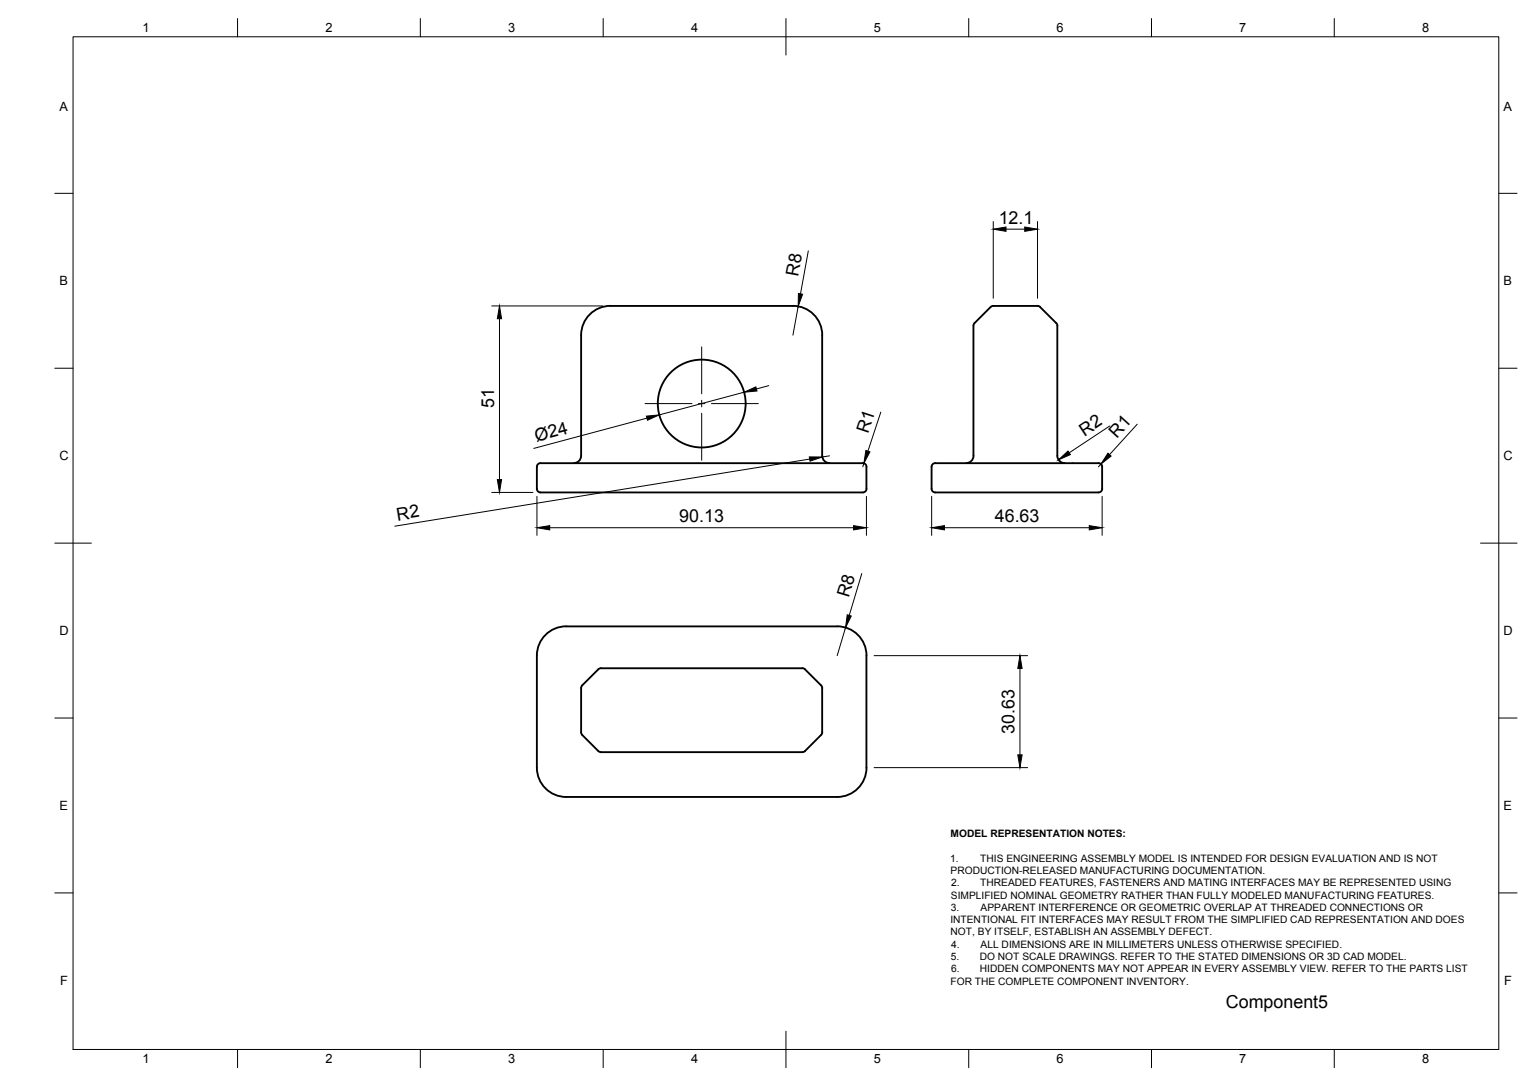
ISO-10303-21;
HEADER;
/* Generated by software containing ST-Developer
 * from STEP Tools, Inc. (www.steptools.com) 
 */

FILE_DESCRIPTION(
/* description */ ('STEP AP214'),
/* implementation_level */ '2;1');

FILE_NAME(
/* name */ 'Component5.step',
/* time_stamp */ '2026-10-06T11:02:40-07:00',
/* author */ (''),
/* organization */ (''),
/* preprocessor_version */ 'ST-DEVELOPER v20.2',
/* originating_system */ 'Autodesk Translation Framework v15.15.0.0',
/* authorisation */ '');

FILE_SCHEMA (('AUTOMOTIVE_DESIGN { 1 0 10303 214 3 1 1 }'));
ENDSEC;

DATA;
#10=MECHANICAL_DESIGN_GEOMETRIC_PRESENTATION_REPRESENTATION('',(#2940),#130910);
#78=CONICAL_SURFACE('',#48628,2.99999999999998,0.78539816339745);
#79=CONICAL_SURFACE('',#48632,2.99999999999998,0.78539816339745);
#80=CONICAL_SURFACE('',#48637,3.00000000000006,0.785398163397453);
#81=CONICAL_SURFACE('',#48641,3.00000000000006,0.785398163397453);
#721=FACE_BOUND('',#15164,.T.);
#722=FACE_BOUND('',#15172,.T.);
#723=FACE_BOUND('',#15175,.T.);
#2924=SHAPE_REPRESENTATION_RELATIONSHIP('SRR','None',#130946,#2932);
#2932=ADVANCED_BREP_SHAPE_REPRESENTATION('',(#2946),#130906);
#2940=STYLED_ITEM('',(#130991),#2946);
#2946=MANIFOLD_SOLID_BREP('Body1',#45456);
#3618=PLANE('',#48578);
#3619=PLANE('',#48591);
#3620=PLANE('',#48592);
#3621=PLANE('',#48593);
#3622=PLANE('',#48594);
#3623=PLANE('',#48595);
#3624=PLANE('',#48600);
#3625=PLANE('',#48601);
#3626=PLANE('',#48604);
#3627=PLANE('',#48605);
#3628=PLANE('',#48608);
#3629=PLANE('',#48627);
#3630=PLANE('',#48631);
#3631=PLANE('',#48635);
#3632=PLANE('',#48636);
#3633=PLANE('',#48640);
#3634=PLANE('',#48644);
#5186=LINE('',#96931,#6960);
#5187=LINE('',#96938,#6961);
#5188=LINE('',#96942,#6962);
#5189=LINE('',#96946,#6963);
#5190=LINE('',#96949,#6964);
#5191=LINE('',#96952,#6965);
#5192=LINE('',#96956,#6966);
#5193=LINE('',#96960,#6967);
#5194=LINE('',#96964,#6968);
#5195=LINE('',#96968,#6969);
#5196=LINE('',#96972,#6970);
#5197=LINE('',#96976,#6971);
#5198=LINE('',#96980,#6972);
#5199=LINE('',#96985,#6973);
#5200=LINE('',#96987,#6974);
#5201=LINE('',#96989,#6975);
#5202=LINE('',#96990,#6976);
#5203=LINE('',#96994,#6977);
#5204=LINE('',#96996,#6978);
#5205=LINE('',#96998,#6979);
#5206=LINE('',#96999,#6980);
#5207=LINE('',#97003,#6981);
#5208=LINE('',#97005,#6982);
#5209=LINE('',#97007,#6983);
#5210=LINE('',#97008,#6984);
#5211=LINE('',#97012,#6985);
#5212=LINE('',#97014,#6986);
#5213=LINE('',#97016,#6987);
#5214=LINE('',#97017,#6988);
#5215=LINE('',#97023,#6989);
#5216=LINE('',#97027,#6990);
#5217=LINE('',#97031,#6991);
#5218=LINE('',#97034,#6992);
#5219=LINE('',#97038,#6993);
#5220=LINE('',#97040,#6994);
#5221=LINE('',#97042,#6995);
#5222=LINE('',#97043,#6996);
#5223=LINE('',#97047,#6997);
#5224=LINE('',#97049,#6998);
#5225=LINE('',#97051,#6999);
#5226=LINE('',#97055,#7000);
#5227=LINE('',#97060,#7001);
#5228=LINE('',#97062,#7002);
#5229=LINE('',#97064,#7003);
#5230=LINE('',#97065,#7004);
#5231=LINE('',#97069,#7005);
#5232=LINE('',#97071,#7006);
#5233=LINE('',#97073,#7007);
#5234=LINE('',#97077,#7008);
#5235=LINE('',#97082,#7009);
#5236=LINE('',#97084,#7010);
#5237=LINE('',#97086,#7011);
#5238=LINE('',#97087,#7012);
#5239=LINE('',#97109,#7013);
#5240=LINE('',#97111,#7014);
#5241=LINE('',#97113,#7015);
#5242=LINE('',#97114,#7016);
#5243=LINE('',#97118,#7017);
#5244=LINE('',#97124,#7018);
#5245=LINE('',#97125,#7019);
#5246=LINE('',#97126,#7020);
#5247=LINE('',#97130,#7021);
#5248=LINE('',#97135,#7022);
#5249=LINE('',#97137,#7023);
#5250=LINE('',#97138,#7024);
#5251=LINE('',#97142,#7025);
#5252=LINE('',#97144,#7026);
#5253=LINE('',#97146,#7027);
#5254=LINE('',#97147,#7028);
#5255=LINE('',#97151,#7029);
#5256=LINE('',#97157,#7030);
#5257=LINE('',#97158,#7031);
#5258=LINE('',#97159,#7032);
#5259=LINE('',#97163,#7033);
#5260=LINE('',#97168,#7034);
#5261=LINE('',#97170,#7035);
#5262=LINE('',#97171,#7036);
#6960=VECTOR('',#58531,12.);
#6961=VECTOR('',#58538,1000.);
#6962=VECTOR('',#58541,1000.);
#6963=VECTOR('',#58544,1000.);
#6964=VECTOR('',#58547,1000.);
#6965=VECTOR('',#58548,1000.);
#6966=VECTOR('',#58551,1000.);
#6967=VECTOR('',#58554,1000.);
#6968=VECTOR('',#58557,1000.);
#6969=VECTOR('',#58560,1000.);
#6970=VECTOR('',#58563,1000.);
#6971=VECTOR('',#58566,1000.);
#6972=VECTOR('',#58569,1000.);
#6973=VECTOR('',#58574,1000.);
#6974=VECTOR('',#58575,1000.);
#6975=VECTOR('',#58576,1000.);
#6976=VECTOR('',#58577,1000.);
#6977=VECTOR('',#58580,1000.);
#6978=VECTOR('',#58581,1000.);
#6979=VECTOR('',#58582,1000.);
#6980=VECTOR('',#58583,1000.);
#6981=VECTOR('',#58586,1000.);
#6982=VECTOR('',#58587,1000.);
#6983=VECTOR('',#58588,1000.);
#6984=VECTOR('',#58589,1000.);
#6985=VECTOR('',#58592,1000.);
#6986=VECTOR('',#58593,1000.);
#6987=VECTOR('',#58594,1000.);
#6988=VECTOR('',#58595,1000.);
#6989=VECTOR('',#58600,1000.);
#6990=VECTOR('',#58603,1000.);
#6991=VECTOR('',#58606,1000.);
#6992=VECTOR('',#58609,1000.);
#6993=VECTOR('',#58612,1000.);
#6994=VECTOR('',#58613,1000.);
#6995=VECTOR('',#58614,1000.);
#6996=VECTOR('',#58615,1000.);
#6997=VECTOR('',#58618,1000.);
#6998=VECTOR('',#58619,1000.);
#6999=VECTOR('',#58620,1000.);
#7000=VECTOR('',#58623,1000.);
#7001=VECTOR('',#58628,1000.);
#7002=VECTOR('',#58629,1000.);
#7003=VECTOR('',#58630,1000.);
#7004=VECTOR('',#58631,1000.);
#7005=VECTOR('',#58634,1000.);
#7006=VECTOR('',#58635,1000.);
#7007=VECTOR('',#58636,1000.);
#7008=VECTOR('',#58639,1000.);
#7009=VECTOR('',#58644,1000.);
#7010=VECTOR('',#58645,1000.);
#7011=VECTOR('',#58646,1000.);
#7012=VECTOR('',#58647,1000.);
#7013=VECTOR('',#58686,1000.);
#7014=VECTOR('',#58687,1000.);
#7015=VECTOR('',#58688,1000.);
#7016=VECTOR('',#58689,1000.);
#7017=VECTOR('',#58692,1000.);
#7018=VECTOR('',#58699,1000.);
#7019=VECTOR('',#58700,1000.);
#7020=VECTOR('',#58701,1000.);
#7021=VECTOR('',#58704,1000.);
#7022=VECTOR('',#58711,1000.);
#7023=VECTOR('',#58712,1000.);
#7024=VECTOR('',#58713,1000.);
#7025=VECTOR('',#58716,1000.);
#7026=VECTOR('',#58717,1000.);
#7027=VECTOR('',#58718,1000.);
#7028=VECTOR('',#58719,1000.);
#7029=VECTOR('',#58722,1000.);
#7030=VECTOR('',#58729,1000.);
#7031=VECTOR('',#58730,1000.);
#7032=VECTOR('',#58731,1000.);
#7033=VECTOR('',#58734,1000.);
#7034=VECTOR('',#58741,1000.);
#7035=VECTOR('',#58742,1000.);
#7036=VECTOR('',#58743,1000.);
#8619=CYLINDRICAL_SURFACE('',#48575,12.);
#8620=CYLINDRICAL_SURFACE('',#48609,8.00000000000001);
#8621=CYLINDRICAL_SURFACE('',#48612,8.00000000000001);
#8622=CYLINDRICAL_SURFACE('',#48615,8.);
#8623=CYLINDRICAL_SURFACE('',#48618,8.);
#8624=CYLINDRICAL_SURFACE('',#48621,8.);
#8625=CYLINDRICAL_SURFACE('',#48624,8.);
#8626=CYLINDRICAL_SURFACE('',#48645,1.);
#8627=CYLINDRICAL_SURFACE('',#48652,1.);
#8628=CYLINDRICAL_SURFACE('',#48654,1.);
#8629=CYLINDRICAL_SURFACE('',#48660,1.);
#8630=CYLINDRICAL_SURFACE('',#48661,1.);
#8631=CYLINDRICAL_SURFACE('',#48668,1.);
#8632=CYLINDRICAL_SURFACE('',#48670,1.);
#8633=CYLINDRICAL_SURFACE('',#48676,1.);
#8634=CYLINDRICAL_SURFACE('',#48677,1.);
#8635=CYLINDRICAL_SURFACE('',#48682,1.);
#8636=CYLINDRICAL_SURFACE('',#48686,1.);
#8637=CYLINDRICAL_SURFACE('',#48688,1.);
#8638=CYLINDRICAL_SURFACE('',#48693,1.);
#8639=CYLINDRICAL_SURFACE('',#48697,1.);
#8640=CYLINDRICAL_SURFACE('',#48699,1.);
#8641=CYLINDRICAL_SURFACE('',#48704,1.);
#8642=CYLINDRICAL_SURFACE('',#48708,1.);
#8643=CYLINDRICAL_SURFACE('',#48710,1.);
#8644=CYLINDRICAL_SURFACE('',#48715,1.);
#8645=CYLINDRICAL_SURFACE('',#48719,1.);
#8646=CYLINDRICAL_SURFACE('',#48724,1.99999999999999);
#8647=CYLINDRICAL_SURFACE('',#48726,2.);
#8648=CYLINDRICAL_SURFACE('',#48732,2.);
#8649=CYLINDRICAL_SURFACE('',#48734,1.99999999999999);
#8650=CYLINDRICAL_SURFACE('',#48740,1.99999999999999);
#8651=CYLINDRICAL_SURFACE('',#48742,2.);
#8652=CYLINDRICAL_SURFACE('',#48748,2.);
#8653=CYLINDRICAL_SURFACE('',#48750,1.99999999999999);
#11123=FACE_OUTER_BOUND('',#15162,.T.);
#11124=FACE_OUTER_BOUND('',#15163,.T.);
#11125=FACE_OUTER_BOUND('',#15165,.T.);
#11126=FACE_OUTER_BOUND('',#15166,.T.);
#11127=FACE_OUTER_BOUND('',#15167,.T.);
#11128=FACE_OUTER_BOUND('',#15168,.T.);
#11129=FACE_OUTER_BOUND('',#15169,.T.);
#11130=FACE_OUTER_BOUND('',#15170,.T.);
#11131=FACE_OUTER_BOUND('',#15171,.T.);
#11132=FACE_OUTER_BOUND('',#15173,.T.);
#11133=FACE_OUTER_BOUND('',#15174,.T.);
#11134=FACE_OUTER_BOUND('',#15176,.T.);
#11135=FACE_OUTER_BOUND('',#15177,.T.);
#11136=FACE_OUTER_BOUND('',#15178,.T.);
#11137=FACE_OUTER_BOUND('',#15179,.T.);
#11138=FACE_OUTER_BOUND('',#15180,.T.);
#11139=FACE_OUTER_BOUND('',#15181,.T.);
#11140=FACE_OUTER_BOUND('',#15182,.T.);
#11141=FACE_OUTER_BOUND('',#15183,.T.);
#11142=FACE_OUTER_BOUND('',#15184,.T.);
#11143=FACE_OUTER_BOUND('',#15185,.T.);
#11144=FACE_OUTER_BOUND('',#15186,.T.);
#11145=FACE_OUTER_BOUND('',#15187,.T.);
#11146=FACE_OUTER_BOUND('',#15188,.T.);
#11147=FACE_OUTER_BOUND('',#15189,.T.);
#11148=FACE_OUTER_BOUND('',#15190,.T.);
#11149=FACE_OUTER_BOUND('',#15191,.T.);
#11150=FACE_OUTER_BOUND('',#15192,.T.);
#11151=FACE_OUTER_BOUND('',#15193,.T.);
#11152=FACE_OUTER_BOUND('',#15194,.T.);
#11153=FACE_OUTER_BOUND('',#15195,.T.);
#11154=FACE_OUTER_BOUND('',#15196,.T.);
#11155=FACE_OUTER_BOUND('',#15197,.T.);
#11156=FACE_OUTER_BOUND('',#15198,.T.);
#11157=FACE_OUTER_BOUND('',#15199,.T.);
#11158=FACE_OUTER_BOUND('',#15200,.T.);
#11159=FACE_OUTER_BOUND('',#15201,.T.);
#11160=FACE_OUTER_BOUND('',#15202,.T.);
#11161=FACE_OUTER_BOUND('',#15203,.T.);
#11162=FACE_OUTER_BOUND('',#15204,.T.);
#11163=FACE_OUTER_BOUND('',#15205,.T.);
#11164=FACE_OUTER_BOUND('',#15206,.T.);
#11165=FACE_OUTER_BOUND('',#15207,.T.);
#11166=FACE_OUTER_BOUND('',#15208,.T.);
#11167=FACE_OUTER_BOUND('',#15209,.T.);
#11168=FACE_OUTER_BOUND('',#15210,.T.);
#11169=FACE_OUTER_BOUND('',#15211,.T.);
#11170=FACE_OUTER_BOUND('',#15212,.T.);
#11171=FACE_OUTER_BOUND('',#15213,.T.);
#11172=FACE_OUTER_BOUND('',#15214,.T.);
#11173=FACE_OUTER_BOUND('',#15215,.T.);
#11174=FACE_OUTER_BOUND('',#15216,.T.);
#11175=FACE_OUTER_BOUND('',#15217,.T.);
#11176=FACE_OUTER_BOUND('',#15218,.T.);
#11177=FACE_OUTER_BOUND('',#15219,.T.);
#11178=FACE_OUTER_BOUND('',#15220,.T.);
#11179=FACE_OUTER_BOUND('',#15221,.T.);
#11180=FACE_OUTER_BOUND('',#15222,.T.);
#11181=FACE_OUTER_BOUND('',#15223,.T.);
#11182=FACE_OUTER_BOUND('',#15224,.T.);
#11183=FACE_OUTER_BOUND('',#15225,.T.);
#11184=FACE_OUTER_BOUND('',#15226,.T.);
#11185=FACE_OUTER_BOUND('',#15227,.T.);
#11186=FACE_OUTER_BOUND('',#15228,.T.);
#11187=FACE_OUTER_BOUND('',#15229,.T.);
#11188=FACE_OUTER_BOUND('',#15230,.T.);
#11189=FACE_OUTER_BOUND('',#15231,.T.);
#11190=FACE_OUTER_BOUND('',#15232,.T.);
#11191=FACE_OUTER_BOUND('',#15233,.T.);
#11192=FACE_OUTER_BOUND('',#15234,.T.);
#11193=FACE_OUTER_BOUND('',#15235,.T.);
#11194=FACE_OUTER_BOUND('',#15236,.T.);
#11195=FACE_OUTER_BOUND('',#15237,.T.);
#11196=FACE_OUTER_BOUND('',#15238,.T.);
#11197=FACE_OUTER_BOUND('',#15239,.T.);
#11198=FACE_OUTER_BOUND('',#15240,.T.);
#11199=FACE_OUTER_BOUND('',#15241,.T.);
#11200=FACE_OUTER_BOUND('',#15242,.T.);
#11201=FACE_OUTER_BOUND('',#15243,.T.);
#11202=FACE_OUTER_BOUND('',#15244,.T.);
#15162=EDGE_LOOP('',(#36076,#36077,#36078,#36079));
#15163=EDGE_LOOP('',(#36080,#36081,#36082,#36083,#36084,#36085,#36086,#36087));
#15164=EDGE_LOOP('',(#36088,#36089,#36090,#36091,#36092,#36093,#36094,#36095,
#36096,#36097,#36098,#36099,#36100,#36101,#36102,#36103));
#15165=EDGE_LOOP('',(#36104,#36105,#36106,#36107));
#15166=EDGE_LOOP('',(#36108,#36109,#36110,#36111));
#15167=EDGE_LOOP('',(#36112,#36113,#36114,#36115));
#15168=EDGE_LOOP('',(#36116,#36117,#36118,#36119));
#15169=EDGE_LOOP('',(#36120,#36121,#36122,#36123,#36124,#36125,#36126,#36127));
#15170=EDGE_LOOP('',(#36128,#36129,#36130,#36131));
#15171=EDGE_LOOP('',(#36132,#36133,#36134,#36135,#36136,#36137));
#15172=EDGE_LOOP('',(#36138));
#15173=EDGE_LOOP('',(#36139,#36140,#36141,#36142));
#15174=EDGE_LOOP('',(#36143,#36144,#36145,#36146,#36147,#36148));
#15175=EDGE_LOOP('',(#36149));
#15176=EDGE_LOOP('',(#36150,#36151,#36152,#36153));
#15177=EDGE_LOOP('',(#36154,#36155,#36156,#36157));
#15178=EDGE_LOOP('',(#36158,#36159,#36160,#36161));
#15179=EDGE_LOOP('',(#36162,#36163,#36164,#36165));
#15180=EDGE_LOOP('',(#36166,#36167,#36168,#36169));
#15181=EDGE_LOOP('',(#36170,#36171,#36172,#36173));
#15182=EDGE_LOOP('',(#36174,#36175,#36176,#36177));
#15183=EDGE_LOOP('',(#36178,#36179,#36180,#36181));
#15184=EDGE_LOOP('',(#36182,#36183,#36184,#36185));
#15185=EDGE_LOOP('',(#36186,#36187,#36188,#36189));
#15186=EDGE_LOOP('',(#36190,#36191,#36192,#36193));
#15187=EDGE_LOOP('',(#36194,#36195,#36196,#36197));
#15188=EDGE_LOOP('',(#36198,#36199,#36200,#36201));
#15189=EDGE_LOOP('',(#36202,#36203,#36204,#36205));
#15190=EDGE_LOOP('',(#36206,#36207,#36208,#36209));
#15191=EDGE_LOOP('',(#36210,#36211,#36212,#36213));
#15192=EDGE_LOOP('',(#36214,#36215,#36216,#36217));
#15193=EDGE_LOOP('',(#36218,#36219,#36220,#36221));
#15194=EDGE_LOOP('',(#36222,#36223,#36224,#36225));
#15195=EDGE_LOOP('',(#36226,#36227,#36228,#36229));
#15196=EDGE_LOOP('',(#36230,#36231,#36232,#36233));
#15197=EDGE_LOOP('',(#36234,#36235,#36236,#36237));
#15198=EDGE_LOOP('',(#36238,#36239,#36240,#36241));
#15199=EDGE_LOOP('',(#36242,#36243,#36244,#36245));
#15200=EDGE_LOOP('',(#36246,#36247,#36248,#36249));
#15201=EDGE_LOOP('',(#36250,#36251,#36252,#36253));
#15202=EDGE_LOOP('',(#36254,#36255,#36256,#36257));
#15203=EDGE_LOOP('',(#36258,#36259,#36260,#36261));
#15204=EDGE_LOOP('',(#36262,#36263,#36264,#36265));
#15205=EDGE_LOOP('',(#36266,#36267,#36268,#36269));
#15206=EDGE_LOOP('',(#36270,#36271,#36272,#36273));
#15207=EDGE_LOOP('',(#36274,#36275,#36276,#36277));
#15208=EDGE_LOOP('',(#36278,#36279,#36280,#36281));
#15209=EDGE_LOOP('',(#36282,#36283,#36284,#36285));
#15210=EDGE_LOOP('',(#36286,#36287,#36288,#36289));
#15211=EDGE_LOOP('',(#36290,#36291,#36292,#36293));
#15212=EDGE_LOOP('',(#36294,#36295,#36296,#36297));
#15213=EDGE_LOOP('',(#36298,#36299,#36300,#36301));
#15214=EDGE_LOOP('',(#36302,#36303,#36304,#36305));
#15215=EDGE_LOOP('',(#36306,#36307,#36308,#36309));
#15216=EDGE_LOOP('',(#36310,#36311,#36312,#36313));
#15217=EDGE_LOOP('',(#36314,#36315,#36316,#36317));
#15218=EDGE_LOOP('',(#36318,#36319,#36320,#36321));
#15219=EDGE_LOOP('',(#36322,#36323,#36324,#36325));
#15220=EDGE_LOOP('',(#36326,#36327,#36328,#36329));
#15221=EDGE_LOOP('',(#36330,#36331,#36332,#36333));
#15222=EDGE_LOOP('',(#36334,#36335,#36336,#36337));
#15223=EDGE_LOOP('',(#36338,#36339,#36340,#36341));
#15224=EDGE_LOOP('',(#36342,#36343,#36344,#36345));
#15225=EDGE_LOOP('',(#36346,#36347,#36348,#36349));
#15226=EDGE_LOOP('',(#36350,#36351,#36352,#36353));
#15227=EDGE_LOOP('',(#36354,#36355,#36356,#36357));
#15228=EDGE_LOOP('',(#36358,#36359,#36360,#36361));
#15229=EDGE_LOOP('',(#36362,#36363,#36364,#36365));
#15230=EDGE_LOOP('',(#36366,#36367,#36368,#36369));
#15231=EDGE_LOOP('',(#36370,#36371,#36372,#36373));
#15232=EDGE_LOOP('',(#36374,#36375,#36376,#36377));
#15233=EDGE_LOOP('',(#36378,#36379,#36380,#36381));
#15234=EDGE_LOOP('',(#36382,#36383,#36384,#36385));
#15235=EDGE_LOOP('',(#36386,#36387,#36388,#36389));
#15236=EDGE_LOOP('',(#36390,#36391,#36392,#36393));
#15237=EDGE_LOOP('',(#36394,#36395,#36396,#36397));
#15238=EDGE_LOOP('',(#36398,#36399,#36400,#36401));
#15239=EDGE_LOOP('',(#36402,#36403,#36404,#36405));
#15240=EDGE_LOOP('',(#36406,#36407,#36408,#36409));
#15241=EDGE_LOOP('',(#36410,#36411,#36412,#36413));
#15242=EDGE_LOOP('',(#36414,#36415,#36416,#36417));
#15243=EDGE_LOOP('',(#36418,#36419,#36420,#36421));
#15244=EDGE_LOOP('',(#36422,#36423,#36424,#36425));
#19217=CIRCLE('',#48576,12.);
#19218=CIRCLE('',#48577,12.);
#19219=CIRCLE('',#48579,7.);
#19220=CIRCLE('',#48580,7.);
#19221=CIRCLE('',#48581,7.);
#19222=CIRCLE('',#48582,7.);
#19223=CIRCLE('',#48583,3.);
#19224=CIRCLE('',#48584,3.);
#19225=CIRCLE('',#48585,3.);
#19226=CIRCLE('',#48586,3.);
#19227=CIRCLE('',#48587,3.);
#19228=CIRCLE('',#48588,3.);
#19229=CIRCLE('',#48589,3.);
#19230=CIRCLE('',#48590,3.);
#19231=CIRCLE('',#48596,7.);
#19232=CIRCLE('',#48597,7.);
#19233=CIRCLE('',#48598,7.);
#19234=CIRCLE('',#48599,7.);
#19235=CIRCLE('',#48602,2.58578643762686);
#19236=CIRCLE('',#48603,2.58578643762686);
#19237=CIRCLE('',#48606,2.58578643762694);
#19238=CIRCLE('',#48607,2.58578643762694);
#19239=CIRCLE('',#48610,8.00000000000001);
#19240=CIRCLE('',#48611,8.00000000000001);
#19241=CIRCLE('',#48613,8.00000000000001);
#19242=CIRCLE('',#48614,8.00000000000001);
#19243=CIRCLE('',#48616,8.);
#19244=CIRCLE('',#48617,8.);
#19245=CIRCLE('',#48619,8.);
#19246=CIRCLE('',#48620,8.);
#19247=CIRCLE('',#48622,8.);
#19248=CIRCLE('',#48623,8.);
#19249=CIRCLE('',#48625,8.);
#19250=CIRCLE('',#48626,8.);
#19251=CIRCLE('',#48629,7.70710678118658);
#19252=CIRCLE('',#48630,3.29289321881343);
#19253=CIRCLE('',#48633,7.70710678118658);
#19254=CIRCLE('',#48634,3.29289321881343);
#19255=CIRCLE('',#48638,3.29289321881349);
#19256=CIRCLE('',#48639,7.70710678118658);
#19257=CIRCLE('',#48642,3.29289321881349);
#19258=CIRCLE('',#48643,7.70710678118658);
#19259=CIRCLE('',#48646,1.);
#19260=CIRCLE('',#48647,1.);
#19261=CIRCLE('',#48649,1.);
#19262=CIRCLE('',#48651,1.);
#19263=CIRCLE('',#48653,1.);
#19264=CIRCLE('',#48655,1.);
#19265=CIRCLE('',#48657,1.);
#19266=CIRCLE('',#48659,1.);
#19267=CIRCLE('',#48662,1.);
#19268=CIRCLE('',#48663,1.);
#19269=CIRCLE('',#48665,1.);
#19270=CIRCLE('',#48667,1.);
#19271=CIRCLE('',#48669,1.);
#19272=CIRCLE('',#48671,1.);
#19273=CIRCLE('',#48673,1.);
#19274=CIRCLE('',#48675,1.);
#19275=CIRCLE('',#48678,1.);
#19276=CIRCLE('',#48679,1.);
#19277=CIRCLE('',#48681,1.);
#19278=CIRCLE('',#48683,1.);
#19279=CIRCLE('',#48685,1.);
#19280=CIRCLE('',#48687,1.);
#19281=CIRCLE('',#48689,1.);
#19282=CIRCLE('',#48690,1.);
#19283=CIRCLE('',#48692,1.);
#19284=CIRCLE('',#48694,1.);
#19285=CIRCLE('',#48696,1.);
#19286=CIRCLE('',#48698,1.);
#19287=CIRCLE('',#48700,1.);
#19288=CIRCLE('',#48701,1.);
#19289=CIRCLE('',#48703,1.);
#19290=CIRCLE('',#48705,1.);
#19291=CIRCLE('',#48707,1.);
#19292=CIRCLE('',#48709,1.);
#19293=CIRCLE('',#48711,1.);
#19294=CIRCLE('',#48712,1.);
#19295=CIRCLE('',#48714,1.);
#19296=CIRCLE('',#48716,1.);
#19297=CIRCLE('',#48718,1.);
#19298=CIRCLE('',#48720,1.);
#19299=CIRCLE('',#48722,2.);
#19300=CIRCLE('',#48723,1.99999999999997);
#19301=CIRCLE('',#48725,2.00000000000002);
#19302=CIRCLE('',#48727,2.);
#19303=CIRCLE('',#48729,2.);
#19304=CIRCLE('',#48731,2.00000000000001);
#19305=CIRCLE('',#48733,2.);
#19306=CIRCLE('',#48735,2.00000000000002);
#19307=CIRCLE('',#48737,2.00000000000001);
#19308=CIRCLE('',#48739,2.);
#19309=CIRCLE('',#48741,2.00000000000002);
#19310=CIRCLE('',#48743,2.);
#19311=CIRCLE('',#48745,2.);
#19312=CIRCLE('',#48747,2.00000000000001);
#19313=CIRCLE('',#48749,2.);
#19314=CIRCLE('',#48751,2.00000000000002);
#22513=VERTEX_POINT('',#96928);
#22514=VERTEX_POINT('',#96930);
#22515=VERTEX_POINT('',#96934);
#22516=VERTEX_POINT('',#96935);
#22517=VERTEX_POINT('',#96937);
#22518=VERTEX_POINT('',#96939);
#22519=VERTEX_POINT('',#96941);
#22520=VERTEX_POINT('',#96943);
#22521=VERTEX_POINT('',#96945);
#22522=VERTEX_POINT('',#96947);
#22523=VERTEX_POINT('',#96950);
#22524=VERTEX_POINT('',#96951);
#22525=VERTEX_POINT('',#96953);
#22526=VERTEX_POINT('',#96955);
#22527=VERTEX_POINT('',#96957);
#22528=VERTEX_POINT('',#96959);
#22529=VERTEX_POINT('',#96961);
#22530=VERTEX_POINT('',#96963);
#22531=VERTEX_POINT('',#96965);
#22532=VERTEX_POINT('',#96967);
#22533=VERTEX_POINT('',#96969);
#22534=VERTEX_POINT('',#96971);
#22535=VERTEX_POINT('',#96973);
#22536=VERTEX_POINT('',#96975);
#22537=VERTEX_POINT('',#96977);
#22538=VERTEX_POINT('',#96979);
#22539=VERTEX_POINT('',#96983);
#22540=VERTEX_POINT('',#96984);
#22541=VERTEX_POINT('',#96986);
#22542=VERTEX_POINT('',#96988);
#22543=VERTEX_POINT('',#96992);
#22544=VERTEX_POINT('',#96993);
#22545=VERTEX_POINT('',#96995);
#22546=VERTEX_POINT('',#96997);
#22547=VERTEX_POINT('',#97001);
#22548=VERTEX_POINT('',#97002);
#22549=VERTEX_POINT('',#97004);
#22550=VERTEX_POINT('',#97006);
#22551=VERTEX_POINT('',#97010);
#22552=VERTEX_POINT('',#97011);
#22553=VERTEX_POINT('',#97013);
#22554=VERTEX_POINT('',#97015);
#22555=VERTEX_POINT('',#97019);
#22556=VERTEX_POINT('',#97020);
#22557=VERTEX_POINT('',#97022);
#22558=VERTEX_POINT('',#97024);
#22559=VERTEX_POINT('',#97026);
#22560=VERTEX_POINT('',#97028);
#22561=VERTEX_POINT('',#97030);
#22562=VERTEX_POINT('',#97032);
#22563=VERTEX_POINT('',#97036);
#22564=VERTEX_POINT('',#97037);
#22565=VERTEX_POINT('',#97039);
#22566=VERTEX_POINT('',#97041);
#22567=VERTEX_POINT('',#97045);
#22568=VERTEX_POINT('',#97046);
#22569=VERTEX_POINT('',#97048);
#22570=VERTEX_POINT('',#97050);
#22571=VERTEX_POINT('',#97052);
#22572=VERTEX_POINT('',#97054);
#22573=VERTEX_POINT('',#97058);
#22574=VERTEX_POINT('',#97059);
#22575=VERTEX_POINT('',#97061);
#22576=VERTEX_POINT('',#97063);
#22577=VERTEX_POINT('',#97067);
#22578=VERTEX_POINT('',#97068);
#22579=VERTEX_POINT('',#97070);
#22580=VERTEX_POINT('',#97072);
#22581=VERTEX_POINT('',#97074);
#22582=VERTEX_POINT('',#97076);
#22583=VERTEX_POINT('',#97080);
#22584=VERTEX_POINT('',#97081);
#22585=VERTEX_POINT('',#97083);
#22586=VERTEX_POINT('',#97085);
#22587=VERTEX_POINT('',#97107);
#22588=VERTEX_POINT('',#97108);
#22589=VERTEX_POINT('',#97110);
#22590=VERTEX_POINT('',#97112);
#22591=VERTEX_POINT('',#97116);
#22592=VERTEX_POINT('',#97117);
#22593=VERTEX_POINT('',#97122);
#22594=VERTEX_POINT('',#97123);
#22595=VERTEX_POINT('',#97128);
#22596=VERTEX_POINT('',#97129);
#22597=VERTEX_POINT('',#97134);
#22598=VERTEX_POINT('',#97136);
#22599=VERTEX_POINT('',#97140);
#22600=VERTEX_POINT('',#97141);
#22601=VERTEX_POINT('',#97143);
#22602=VERTEX_POINT('',#97145);
#22603=VERTEX_POINT('',#97149);
#22604=VERTEX_POINT('',#97150);
#22605=VERTEX_POINT('',#97155);
#22606=VERTEX_POINT('',#97156);
#22607=VERTEX_POINT('',#97161);
#22608=VERTEX_POINT('',#97162);
#22609=VERTEX_POINT('',#97167);
#22610=VERTEX_POINT('',#97169);
#27382=EDGE_CURVE('',#22513,#22513,#19217,.T.);
#27383=EDGE_CURVE('',#22513,#22514,#5186,.T.);
#27384=EDGE_CURVE('',#22514,#22514,#19218,.T.);
#27385=EDGE_CURVE('',#22515,#22516,#19219,.T.);
#27386=EDGE_CURVE('',#22516,#22517,#5187,.T.);
#27387=EDGE_CURVE('',#22517,#22518,#19220,.T.);
#27388=EDGE_CURVE('',#22518,#22519,#5188,.T.);
#27389=EDGE_CURVE('',#22519,#22520,#19221,.T.);
#27390=EDGE_CURVE('',#22520,#22521,#5189,.T.);
#27391=EDGE_CURVE('',#22521,#22522,#19222,.T.);
#27392=EDGE_CURVE('',#22522,#22515,#5190,.T.);
#27393=EDGE_CURVE('',#22523,#22524,#5191,.T.);
#27394=EDGE_CURVE('',#22524,#22525,#19223,.T.);
#27395=EDGE_CURVE('',#22525,#22526,#5192,.T.);
#27396=EDGE_CURVE('',#22526,#22527,#19224,.T.);
#27397=EDGE_CURVE('',#22527,#22528,#5193,.T.);
#27398=EDGE_CURVE('',#22528,#22529,#19225,.T.);
#27399=EDGE_CURVE('',#22529,#22530,#5194,.T.);
#27400=EDGE_CURVE('',#22530,#22531,#19226,.T.);
#27401=EDGE_CURVE('',#22531,#22532,#5195,.T.);
#27402=EDGE_CURVE('',#22532,#22533,#19227,.T.);
#27403=EDGE_CURVE('',#22533,#22534,#5196,.T.);
#27404=EDGE_CURVE('',#22534,#22535,#19228,.T.);
#27405=EDGE_CURVE('',#22535,#22536,#5197,.T.);
#27406=EDGE_CURVE('',#22536,#22537,#19229,.T.);
#27407=EDGE_CURVE('',#22537,#22538,#5198,.T.);
#27408=EDGE_CURVE('',#22538,#22523,#19230,.T.);
#27409=EDGE_CURVE('',#22539,#22540,#5199,.T.);
#27410=EDGE_CURVE('',#22540,#22541,#5200,.T.);
#27411=EDGE_CURVE('',#22541,#22542,#5201,.T.);
#27412=EDGE_CURVE('',#22542,#22539,#5202,.T.);
#27413=EDGE_CURVE('',#22543,#22544,#5203,.T.);
#27414=EDGE_CURVE('',#22544,#22545,#5204,.T.);
#27415=EDGE_CURVE('',#22545,#22546,#5205,.T.);
#27416=EDGE_CURVE('',#22546,#22543,#5206,.T.);
#27417=EDGE_CURVE('',#22547,#22548,#5207,.T.);
#27418=EDGE_CURVE('',#22548,#22549,#5208,.T.);
#27419=EDGE_CURVE('',#22549,#22550,#5209,.T.);
#27420=EDGE_CURVE('',#22550,#22547,#5210,.T.);
#27421=EDGE_CURVE('',#22551,#22552,#5211,.T.);
#27422=EDGE_CURVE('',#22552,#22553,#5212,.T.);
#27423=EDGE_CURVE('',#22553,#22554,#5213,.T.);
#27424=EDGE_CURVE('',#22554,#22551,#5214,.T.);
#27425=EDGE_CURVE('',#22555,#22556,#19231,.T.);
#27426=EDGE_CURVE('',#22556,#22557,#5215,.T.);
#27427=EDGE_CURVE('',#22557,#22558,#19232,.T.);
#27428=EDGE_CURVE('',#22558,#22559,#5216,.T.);
#27429=EDGE_CURVE('',#22559,#22560,#19233,.T.);
#27430=EDGE_CURVE('',#22560,#22561,#5217,.T.);
#27431=EDGE_CURVE('',#22561,#22562,#19234,.T.);
#27432=EDGE_CURVE('',#22562,#22555,#5218,.T.);
#27433=EDGE_CURVE('',#22563,#22564,#5219,.T.);
#27434=EDGE_CURVE('',#22564,#22565,#5220,.T.);
#27435=EDGE_CURVE('',#22565,#22566,#5221,.T.);
#27436=EDGE_CURVE('',#22566,#22563,#5222,.T.);
#27437=EDGE_CURVE('',#22567,#22568,#5223,.T.);
#27438=EDGE_CURVE('',#22568,#22569,#5224,.T.);
#27439=EDGE_CURVE('',#22569,#22570,#5225,.T.);
#27440=EDGE_CURVE('',#22570,#22571,#19235,.T.);
#27441=EDGE_CURVE('',#22571,#22572,#5226,.T.);
#27442=EDGE_CURVE('',#22572,#22567,#19236,.T.);
#27443=EDGE_CURVE('',#22573,#22574,#5227,.T.);
#27444=EDGE_CURVE('',#22574,#22575,#5228,.T.);
#27445=EDGE_CURVE('',#22575,#22576,#5229,.T.);
#27446=EDGE_CURVE('',#22576,#22573,#5230,.T.);
#27447=EDGE_CURVE('',#22577,#22578,#5231,.T.);
#27448=EDGE_CURVE('',#22578,#22579,#5232,.T.);
#27449=EDGE_CURVE('',#22579,#22580,#5233,.T.);
#27450=EDGE_CURVE('',#22580,#22581,#19237,.T.);
#27451=EDGE_CURVE('',#22581,#22582,#5234,.T.);
#27452=EDGE_CURVE('',#22582,#22577,#19238,.T.);
#27453=EDGE_CURVE('',#22583,#22584,#5235,.T.);
#27454=EDGE_CURVE('',#22584,#22585,#5236,.T.);
#27455=EDGE_CURVE('',#22585,#22586,#5237,.T.);
#27456=EDGE_CURVE('',#22586,#22583,#5238,.T.);
#27457=EDGE_CURVE('',#22585,#22573,#19239,.T.);
#27458=EDGE_CURVE('',#22576,#22586,#19240,.T.);
#27459=EDGE_CURVE('',#22566,#22584,#19241,.T.);
#27460=EDGE_CURVE('',#22583,#22563,#19242,.T.);
#27461=EDGE_CURVE('',#22549,#22552,#19243,.T.);
#27462=EDGE_CURVE('',#22551,#22550,#19244,.T.);
#27463=EDGE_CURVE('',#22545,#22548,#19245,.T.);
#27464=EDGE_CURVE('',#22547,#22546,#19246,.T.);
#27465=EDGE_CURVE('',#22541,#22544,#19247,.T.);
#27466=EDGE_CURVE('',#22543,#22542,#19248,.T.);
#27467=EDGE_CURVE('',#22553,#22540,#19249,.T.);
#27468=EDGE_CURVE('',#22539,#22554,#19250,.T.);
#27469=EDGE_CURVE('',#22587,#22588,#5239,.T.);
#27470=EDGE_CURVE('',#22588,#22589,#5240,.T.);
#27471=EDGE_CURVE('',#22589,#22590,#5241,.T.);
#27472=EDGE_CURVE('',#22587,#22590,#5242,.T.);
#27473=EDGE_CURVE('',#22591,#22592,#5243,.T.);
#27474=EDGE_CURVE('',#22591,#22587,#19251,.T.);
#27475=EDGE_CURVE('',#22590,#22592,#19252,.T.);
#27476=EDGE_CURVE('',#22593,#22594,#5244,.T.);
#27477=EDGE_CURVE('',#22593,#22591,#5245,.T.);
#27478=EDGE_CURVE('',#22592,#22594,#5246,.T.);
#27479=EDGE_CURVE('',#22595,#22596,#5247,.T.);
#27480=EDGE_CURVE('',#22595,#22593,#19253,.T.);
#27481=EDGE_CURVE('',#22594,#22596,#19254,.T.);
#27482=EDGE_CURVE('',#22596,#22597,#5248,.T.);
#27483=EDGE_CURVE('',#22597,#22598,#5249,.T.);
#27484=EDGE_CURVE('',#22598,#22595,#5250,.T.);
#27485=EDGE_CURVE('',#22599,#22600,#5251,.T.);
#27486=EDGE_CURVE('',#22600,#22601,#5252,.T.);
#27487=EDGE_CURVE('',#22601,#22602,#5253,.T.);
#27488=EDGE_CURVE('',#22599,#22602,#5254,.T.);
#27489=EDGE_CURVE('',#22603,#22604,#5255,.T.);
#27490=EDGE_CURVE('',#22603,#22599,#19255,.T.);
#27491=EDGE_CURVE('',#22602,#22604,#19256,.T.);
#27492=EDGE_CURVE('',#22605,#22606,#5256,.T.);
#27493=EDGE_CURVE('',#22605,#22603,#5257,.T.);
#27494=EDGE_CURVE('',#22604,#22606,#5258,.T.);
#27495=EDGE_CURVE('',#22607,#22608,#5259,.T.);
#27496=EDGE_CURVE('',#22607,#22605,#19257,.T.);
#27497=EDGE_CURVE('',#22606,#22608,#19258,.T.);
#27498=EDGE_CURVE('',#22608,#22609,#5260,.T.);
#27499=EDGE_CURVE('',#22609,#22610,#5261,.T.);
#27500=EDGE_CURVE('',#22610,#22607,#5262,.T.);
#27501=EDGE_CURVE('',#22549,#22560,#19259,.T.);
#27502=EDGE_CURVE('',#22561,#22548,#19260,.T.);
#27503=EDGE_CURVE('',#22562,#22545,#19261,.T.);
#27504=EDGE_CURVE('',#22552,#22559,#19262,.T.);
#27505=EDGE_CURVE('',#22555,#22544,#19263,.T.);
#27506=EDGE_CURVE('',#22553,#22558,#19264,.T.);
#27507=EDGE_CURVE('',#22556,#22541,#19265,.T.);
#27508=EDGE_CURVE('',#22540,#22557,#19266,.T.);
#27509=EDGE_CURVE('',#22521,#22546,#19267,.T.);
#27510=EDGE_CURVE('',#22543,#22520,#19268,.T.);
#27511=EDGE_CURVE('',#22542,#22519,#19269,.T.);
#27512=EDGE_CURVE('',#22522,#22547,#19270,.T.);
#27513=EDGE_CURVE('',#22539,#22518,#19271,.T.);
#27514=EDGE_CURVE('',#22515,#22550,#19272,.T.);
#27515=EDGE_CURVE('',#22554,#22517,#19273,.T.);
#27516=EDGE_CURVE('',#22516,#22551,#19274,.T.);
#27517=EDGE_CURVE('',#22598,#22574,#19275,.T.);
#27518=EDGE_CURVE('',#22595,#22573,#19276,.T.);
#27519=EDGE_CURVE('',#22593,#22585,#19277,.T.);
#27520=EDGE_CURVE('',#22591,#22584,#19278,.T.);
#27521=EDGE_CURVE('',#22587,#22566,#19279,.T.);
#27522=EDGE_CURVE('',#22565,#22588,#19280,.T.);
#27523=EDGE_CURVE('',#22589,#22568,#19281,.T.);
#27524=EDGE_CURVE('',#22590,#22567,#19282,.T.);
#27525=EDGE_CURVE('',#22592,#22572,#19283,.T.);
#27526=EDGE_CURVE('',#22594,#22571,#19284,.T.);
#27527=EDGE_CURVE('',#22596,#22570,#19285,.T.);
#27528=EDGE_CURVE('',#22569,#22597,#19286,.T.);
#27529=EDGE_CURVE('',#22610,#22578,#19287,.T.);
#27530=EDGE_CURVE('',#22607,#22577,#19288,.T.);
#27531=EDGE_CURVE('',#22605,#22582,#19289,.T.);
#27532=EDGE_CURVE('',#22603,#22581,#19290,.T.);
#27533=EDGE_CURVE('',#22599,#22580,#19291,.T.);
#27534=EDGE_CURVE('',#22579,#22600,#19292,.T.);
#27535=EDGE_CURVE('',#22601,#22564,#19293,.T.);
#27536=EDGE_CURVE('',#22602,#22563,#19294,.T.);
#27537=EDGE_CURVE('',#22604,#22583,#19295,.T.);
#27538=EDGE_CURVE('',#22606,#22586,#19296,.T.);
#27539=EDGE_CURVE('',#22608,#22576,#19297,.T.);
#27540=EDGE_CURVE('',#22575,#22609,#19298,.T.);
#27541=EDGE_CURVE('',#22574,#22532,#19299,.T.);
#27542=EDGE_CURVE('',#22533,#22598,#19300,.T.);
#27543=EDGE_CURVE('',#22534,#22597,#19301,.T.);
#27544=EDGE_CURVE('',#22575,#22531,#19302,.T.);
#27545=EDGE_CURVE('',#22535,#22569,#19303,.T.);
#27546=EDGE_CURVE('',#22609,#22530,#19304,.T.);
#27547=EDGE_CURVE('',#22536,#22568,#19305,.T.);
#27548=EDGE_CURVE('',#22610,#22529,#19306,.T.);
#27549=EDGE_CURVE('',#22537,#22589,#19307,.T.);
#27550=EDGE_CURVE('',#22578,#22528,#19308,.T.);
#27551=EDGE_CURVE('',#22538,#22588,#19309,.T.);
#27552=EDGE_CURVE('',#22579,#22527,#19310,.T.);
#27553=EDGE_CURVE('',#22523,#22565,#19311,.T.);
#27554=EDGE_CURVE('',#22600,#22526,#19312,.T.);
#27555=EDGE_CURVE('',#22524,#22564,#19313,.T.);
#27556=EDGE_CURVE('',#22601,#22525,#19314,.T.);
#36076=ORIENTED_EDGE('',*,*,#27382,.F.);
#36077=ORIENTED_EDGE('',*,*,#27383,.T.);
#36078=ORIENTED_EDGE('',*,*,#27384,.T.);
#36079=ORIENTED_EDGE('',*,*,#27383,.F.);
#36080=ORIENTED_EDGE('',*,*,#27385,.T.);
#36081=ORIENTED_EDGE('',*,*,#27386,.T.);
#36082=ORIENTED_EDGE('',*,*,#27387,.T.);
#36083=ORIENTED_EDGE('',*,*,#27388,.T.);
#36084=ORIENTED_EDGE('',*,*,#27389,.T.);
#36085=ORIENTED_EDGE('',*,*,#27390,.T.);
#36086=ORIENTED_EDGE('',*,*,#27391,.T.);
#36087=ORIENTED_EDGE('',*,*,#27392,.T.);
#36088=ORIENTED_EDGE('',*,*,#27393,.T.);
#36089=ORIENTED_EDGE('',*,*,#27394,.T.);
#36090=ORIENTED_EDGE('',*,*,#27395,.T.);
#36091=ORIENTED_EDGE('',*,*,#27396,.T.);
#36092=ORIENTED_EDGE('',*,*,#27397,.T.);
#36093=ORIENTED_EDGE('',*,*,#27398,.T.);
#36094=ORIENTED_EDGE('',*,*,#27399,.T.);
#36095=ORIENTED_EDGE('',*,*,#27400,.T.);
#36096=ORIENTED_EDGE('',*,*,#27401,.T.);
#36097=ORIENTED_EDGE('',*,*,#27402,.T.);
#36098=ORIENTED_EDGE('',*,*,#27403,.T.);
#36099=ORIENTED_EDGE('',*,*,#27404,.T.);
#36100=ORIENTED_EDGE('',*,*,#27405,.T.);
#36101=ORIENTED_EDGE('',*,*,#27406,.T.);
#36102=ORIENTED_EDGE('',*,*,#27407,.T.);
#36103=ORIENTED_EDGE('',*,*,#27408,.T.);
#36104=ORIENTED_EDGE('',*,*,#27409,.T.);
#36105=ORIENTED_EDGE('',*,*,#27410,.T.);
#36106=ORIENTED_EDGE('',*,*,#27411,.T.);
#36107=ORIENTED_EDGE('',*,*,#27412,.T.);
#36108=ORIENTED_EDGE('',*,*,#27413,.T.);
#36109=ORIENTED_EDGE('',*,*,#27414,.T.);
#36110=ORIENTED_EDGE('',*,*,#27415,.T.);
#36111=ORIENTED_EDGE('',*,*,#27416,.T.);
#36112=ORIENTED_EDGE('',*,*,#27417,.T.);
#36113=ORIENTED_EDGE('',*,*,#27418,.T.);
#36114=ORIENTED_EDGE('',*,*,#27419,.T.);
#36115=ORIENTED_EDGE('',*,*,#27420,.T.);
#36116=ORIENTED_EDGE('',*,*,#27421,.T.);
#36117=ORIENTED_EDGE('',*,*,#27422,.T.);
#36118=ORIENTED_EDGE('',*,*,#27423,.T.);
#36119=ORIENTED_EDGE('',*,*,#27424,.T.);
#36120=ORIENTED_EDGE('',*,*,#27425,.T.);
#36121=ORIENTED_EDGE('',*,*,#27426,.T.);
#36122=ORIENTED_EDGE('',*,*,#27427,.T.);
#36123=ORIENTED_EDGE('',*,*,#27428,.T.);
#36124=ORIENTED_EDGE('',*,*,#27429,.T.);
#36125=ORIENTED_EDGE('',*,*,#27430,.T.);
#36126=ORIENTED_EDGE('',*,*,#27431,.T.);
#36127=ORIENTED_EDGE('',*,*,#27432,.T.);
#36128=ORIENTED_EDGE('',*,*,#27433,.T.);
#36129=ORIENTED_EDGE('',*,*,#27434,.T.);
#36130=ORIENTED_EDGE('',*,*,#27435,.T.);
#36131=ORIENTED_EDGE('',*,*,#27436,.T.);
#36132=ORIENTED_EDGE('',*,*,#27437,.T.);
#36133=ORIENTED_EDGE('',*,*,#27438,.T.);
#36134=ORIENTED_EDGE('',*,*,#27439,.T.);
#36135=ORIENTED_EDGE('',*,*,#27440,.T.);
#36136=ORIENTED_EDGE('',*,*,#27441,.T.);
#36137=ORIENTED_EDGE('',*,*,#27442,.T.);
#36138=ORIENTED_EDGE('',*,*,#27382,.T.);
#36139=ORIENTED_EDGE('',*,*,#27443,.T.);
#36140=ORIENTED_EDGE('',*,*,#27444,.T.);
#36141=ORIENTED_EDGE('',*,*,#27445,.T.);
#36142=ORIENTED_EDGE('',*,*,#27446,.T.);
#36143=ORIENTED_EDGE('',*,*,#27447,.T.);
#36144=ORIENTED_EDGE('',*,*,#27448,.T.);
#36145=ORIENTED_EDGE('',*,*,#27449,.T.);
#36146=ORIENTED_EDGE('',*,*,#27450,.T.);
#36147=ORIENTED_EDGE('',*,*,#27451,.T.);
#36148=ORIENTED_EDGE('',*,*,#27452,.T.);
#36149=ORIENTED_EDGE('',*,*,#27384,.F.);
#36150=ORIENTED_EDGE('',*,*,#27453,.T.);
#36151=ORIENTED_EDGE('',*,*,#27454,.T.);
#36152=ORIENTED_EDGE('',*,*,#27455,.T.);
#36153=ORIENTED_EDGE('',*,*,#27456,.T.);
#36154=ORIENTED_EDGE('',*,*,#27455,.F.);
#36155=ORIENTED_EDGE('',*,*,#27457,.T.);
#36156=ORIENTED_EDGE('',*,*,#27446,.F.);
#36157=ORIENTED_EDGE('',*,*,#27458,.T.);
#36158=ORIENTED_EDGE('',*,*,#27436,.F.);
#36159=ORIENTED_EDGE('',*,*,#27459,.T.);
#36160=ORIENTED_EDGE('',*,*,#27453,.F.);
#36161=ORIENTED_EDGE('',*,*,#27460,.T.);
#36162=ORIENTED_EDGE('',*,*,#27419,.F.);
#36163=ORIENTED_EDGE('',*,*,#27461,.T.);
#36164=ORIENTED_EDGE('',*,*,#27421,.F.);
#36165=ORIENTED_EDGE('',*,*,#27462,.T.);
#36166=ORIENTED_EDGE('',*,*,#27415,.F.);
#36167=ORIENTED_EDGE('',*,*,#27463,.T.);
#36168=ORIENTED_EDGE('',*,*,#27417,.F.);
#36169=ORIENTED_EDGE('',*,*,#27464,.T.);
#36170=ORIENTED_EDGE('',*,*,#27411,.F.);
#36171=ORIENTED_EDGE('',*,*,#27465,.T.);
#36172=ORIENTED_EDGE('',*,*,#27413,.F.);
#36173=ORIENTED_EDGE('',*,*,#27466,.T.);
#36174=ORIENTED_EDGE('',*,*,#27423,.F.);
#36175=ORIENTED_EDGE('',*,*,#27467,.T.);
#36176=ORIENTED_EDGE('',*,*,#27409,.F.);
#36177=ORIENTED_EDGE('',*,*,#27468,.T.);
#36178=ORIENTED_EDGE('',*,*,#27469,.T.);
#36179=ORIENTED_EDGE('',*,*,#27470,.T.);
#36180=ORIENTED_EDGE('',*,*,#27471,.T.);
#36181=ORIENTED_EDGE('',*,*,#27472,.F.);
#36182=ORIENTED_EDGE('',*,*,#27473,.F.);
#36183=ORIENTED_EDGE('',*,*,#27474,.T.);
#36184=ORIENTED_EDGE('',*,*,#27472,.T.);
#36185=ORIENTED_EDGE('',*,*,#27475,.T.);
#36186=ORIENTED_EDGE('',*,*,#27476,.F.);
#36187=ORIENTED_EDGE('',*,*,#27477,.T.);
#36188=ORIENTED_EDGE('',*,*,#27473,.T.);
#36189=ORIENTED_EDGE('',*,*,#27478,.T.);
#36190=ORIENTED_EDGE('',*,*,#27479,.F.);
#36191=ORIENTED_EDGE('',*,*,#27480,.T.);
#36192=ORIENTED_EDGE('',*,*,#27476,.T.);
#36193=ORIENTED_EDGE('',*,*,#27481,.T.);
#36194=ORIENTED_EDGE('',*,*,#27482,.T.);
#36195=ORIENTED_EDGE('',*,*,#27483,.T.);
#36196=ORIENTED_EDGE('',*,*,#27484,.T.);
#36197=ORIENTED_EDGE('',*,*,#27479,.T.);
#36198=ORIENTED_EDGE('',*,*,#27485,.T.);
#36199=ORIENTED_EDGE('',*,*,#27486,.T.);
#36200=ORIENTED_EDGE('',*,*,#27487,.T.);
#36201=ORIENTED_EDGE('',*,*,#27488,.F.);
#36202=ORIENTED_EDGE('',*,*,#27489,.F.);
#36203=ORIENTED_EDGE('',*,*,#27490,.T.);
#36204=ORIENTED_EDGE('',*,*,#27488,.T.);
#36205=ORIENTED_EDGE('',*,*,#27491,.T.);
#36206=ORIENTED_EDGE('',*,*,#27492,.F.);
#36207=ORIENTED_EDGE('',*,*,#27493,.T.);
#36208=ORIENTED_EDGE('',*,*,#27489,.T.);
#36209=ORIENTED_EDGE('',*,*,#27494,.T.);
#36210=ORIENTED_EDGE('',*,*,#27495,.F.);
#36211=ORIENTED_EDGE('',*,*,#27496,.T.);
#36212=ORIENTED_EDGE('',*,*,#27492,.T.);
#36213=ORIENTED_EDGE('',*,*,#27497,.T.);
#36214=ORIENTED_EDGE('',*,*,#27498,.T.);
#36215=ORIENTED_EDGE('',*,*,#27499,.T.);
#36216=ORIENTED_EDGE('',*,*,#27500,.T.);
#36217=ORIENTED_EDGE('',*,*,#27495,.T.);
#36218=ORIENTED_EDGE('',*,*,#27501,.F.);
#36219=ORIENTED_EDGE('',*,*,#27418,.F.);
#36220=ORIENTED_EDGE('',*,*,#27502,.F.);
#36221=ORIENTED_EDGE('',*,*,#27430,.F.);
#36222=ORIENTED_EDGE('',*,*,#27502,.T.);
#36223=ORIENTED_EDGE('',*,*,#27463,.F.);
#36224=ORIENTED_EDGE('',*,*,#27503,.F.);
#36225=ORIENTED_EDGE('',*,*,#27431,.F.);
#36226=ORIENTED_EDGE('',*,*,#27501,.T.);
#36227=ORIENTED_EDGE('',*,*,#27429,.F.);
#36228=ORIENTED_EDGE('',*,*,#27504,.F.);
#36229=ORIENTED_EDGE('',*,*,#27461,.F.);
#36230=ORIENTED_EDGE('',*,*,#27503,.T.);
#36231=ORIENTED_EDGE('',*,*,#27414,.F.);
#36232=ORIENTED_EDGE('',*,*,#27505,.F.);
#36233=ORIENTED_EDGE('',*,*,#27432,.F.);
#36234=ORIENTED_EDGE('',*,*,#27504,.T.);
#36235=ORIENTED_EDGE('',*,*,#27428,.F.);
#36236=ORIENTED_EDGE('',*,*,#27506,.F.);
#36237=ORIENTED_EDGE('',*,*,#27422,.F.);
#36238=ORIENTED_EDGE('',*,*,#27505,.T.);
#36239=ORIENTED_EDGE('',*,*,#27465,.F.);
#36240=ORIENTED_EDGE('',*,*,#27507,.F.);
#36241=ORIENTED_EDGE('',*,*,#27425,.F.);
#36242=ORIENTED_EDGE('',*,*,#27506,.T.);
#36243=ORIENTED_EDGE('',*,*,#27427,.F.);
#36244=ORIENTED_EDGE('',*,*,#27508,.F.);
#36245=ORIENTED_EDGE('',*,*,#27467,.F.);
#36246=ORIENTED_EDGE('',*,*,#27507,.T.);
#36247=ORIENTED_EDGE('',*,*,#27410,.F.);
#36248=ORIENTED_EDGE('',*,*,#27508,.T.);
#36249=ORIENTED_EDGE('',*,*,#27426,.F.);
#36250=ORIENTED_EDGE('',*,*,#27509,.F.);
#36251=ORIENTED_EDGE('',*,*,#27390,.F.);
#36252=ORIENTED_EDGE('',*,*,#27510,.F.);
#36253=ORIENTED_EDGE('',*,*,#27416,.F.);
#36254=ORIENTED_EDGE('',*,*,#27510,.T.);
#36255=ORIENTED_EDGE('',*,*,#27389,.F.);
#36256=ORIENTED_EDGE('',*,*,#27511,.F.);
#36257=ORIENTED_EDGE('',*,*,#27466,.F.);
#36258=ORIENTED_EDGE('',*,*,#27509,.T.);
#36259=ORIENTED_EDGE('',*,*,#27464,.F.);
#36260=ORIENTED_EDGE('',*,*,#27512,.F.);
#36261=ORIENTED_EDGE('',*,*,#27391,.F.);
#36262=ORIENTED_EDGE('',*,*,#27511,.T.);
#36263=ORIENTED_EDGE('',*,*,#27388,.F.);
#36264=ORIENTED_EDGE('',*,*,#27513,.F.);
#36265=ORIENTED_EDGE('',*,*,#27412,.F.);
#36266=ORIENTED_EDGE('',*,*,#27512,.T.);
#36267=ORIENTED_EDGE('',*,*,#27420,.F.);
#36268=ORIENTED_EDGE('',*,*,#27514,.F.);
#36269=ORIENTED_EDGE('',*,*,#27392,.F.);
#36270=ORIENTED_EDGE('',*,*,#27513,.T.);
#36271=ORIENTED_EDGE('',*,*,#27387,.F.);
#36272=ORIENTED_EDGE('',*,*,#27515,.F.);
#36273=ORIENTED_EDGE('',*,*,#27468,.F.);
#36274=ORIENTED_EDGE('',*,*,#27514,.T.);
#36275=ORIENTED_EDGE('',*,*,#27462,.F.);
#36276=ORIENTED_EDGE('',*,*,#27516,.F.);
#36277=ORIENTED_EDGE('',*,*,#27385,.F.);
#36278=ORIENTED_EDGE('',*,*,#27515,.T.);
#36279=ORIENTED_EDGE('',*,*,#27386,.F.);
#36280=ORIENTED_EDGE('',*,*,#27516,.T.);
#36281=ORIENTED_EDGE('',*,*,#27424,.F.);
#36282=ORIENTED_EDGE('',*,*,#27484,.F.);
#36283=ORIENTED_EDGE('',*,*,#27517,.T.);
#36284=ORIENTED_EDGE('',*,*,#27443,.F.);
#36285=ORIENTED_EDGE('',*,*,#27518,.F.);
#36286=ORIENTED_EDGE('',*,*,#27518,.T.);
#36287=ORIENTED_EDGE('',*,*,#27457,.F.);
#36288=ORIENTED_EDGE('',*,*,#27519,.F.);
#36289=ORIENTED_EDGE('',*,*,#27480,.F.);
#36290=ORIENTED_EDGE('',*,*,#27519,.T.);
#36291=ORIENTED_EDGE('',*,*,#27454,.F.);
#36292=ORIENTED_EDGE('',*,*,#27520,.F.);
#36293=ORIENTED_EDGE('',*,*,#27477,.F.);
#36294=ORIENTED_EDGE('',*,*,#27520,.T.);
#36295=ORIENTED_EDGE('',*,*,#27459,.F.);
#36296=ORIENTED_EDGE('',*,*,#27521,.F.);
#36297=ORIENTED_EDGE('',*,*,#27474,.F.);
#36298=ORIENTED_EDGE('',*,*,#27435,.F.);
#36299=ORIENTED_EDGE('',*,*,#27522,.T.);
#36300=ORIENTED_EDGE('',*,*,#27469,.F.);
#36301=ORIENTED_EDGE('',*,*,#27521,.T.);
#36302=ORIENTED_EDGE('',*,*,#27471,.F.);
#36303=ORIENTED_EDGE('',*,*,#27523,.T.);
#36304=ORIENTED_EDGE('',*,*,#27437,.F.);
#36305=ORIENTED_EDGE('',*,*,#27524,.F.);
#36306=ORIENTED_EDGE('',*,*,#27524,.T.);
#36307=ORIENTED_EDGE('',*,*,#27442,.F.);
#36308=ORIENTED_EDGE('',*,*,#27525,.F.);
#36309=ORIENTED_EDGE('',*,*,#27475,.F.);
#36310=ORIENTED_EDGE('',*,*,#27525,.T.);
#36311=ORIENTED_EDGE('',*,*,#27441,.F.);
#36312=ORIENTED_EDGE('',*,*,#27526,.F.);
#36313=ORIENTED_EDGE('',*,*,#27478,.F.);
#36314=ORIENTED_EDGE('',*,*,#27526,.T.);
#36315=ORIENTED_EDGE('',*,*,#27440,.F.);
#36316=ORIENTED_EDGE('',*,*,#27527,.F.);
#36317=ORIENTED_EDGE('',*,*,#27481,.F.);
#36318=ORIENTED_EDGE('',*,*,#27439,.F.);
#36319=ORIENTED_EDGE('',*,*,#27528,.T.);
#36320=ORIENTED_EDGE('',*,*,#27482,.F.);
#36321=ORIENTED_EDGE('',*,*,#27527,.T.);
#36322=ORIENTED_EDGE('',*,*,#27500,.F.);
#36323=ORIENTED_EDGE('',*,*,#27529,.T.);
#36324=ORIENTED_EDGE('',*,*,#27447,.F.);
#36325=ORIENTED_EDGE('',*,*,#27530,.F.);
#36326=ORIENTED_EDGE('',*,*,#27530,.T.);
#36327=ORIENTED_EDGE('',*,*,#27452,.F.);
#36328=ORIENTED_EDGE('',*,*,#27531,.F.);
#36329=ORIENTED_EDGE('',*,*,#27496,.F.);
#36330=ORIENTED_EDGE('',*,*,#27531,.T.);
#36331=ORIENTED_EDGE('',*,*,#27451,.F.);
#36332=ORIENTED_EDGE('',*,*,#27532,.F.);
#36333=ORIENTED_EDGE('',*,*,#27493,.F.);
#36334=ORIENTED_EDGE('',*,*,#27532,.T.);
#36335=ORIENTED_EDGE('',*,*,#27450,.F.);
#36336=ORIENTED_EDGE('',*,*,#27533,.F.);
#36337=ORIENTED_EDGE('',*,*,#27490,.F.);
#36338=ORIENTED_EDGE('',*,*,#27449,.F.);
#36339=ORIENTED_EDGE('',*,*,#27534,.T.);
#36340=ORIENTED_EDGE('',*,*,#27485,.F.);
#36341=ORIENTED_EDGE('',*,*,#27533,.T.);
#36342=ORIENTED_EDGE('',*,*,#27487,.F.);
#36343=ORIENTED_EDGE('',*,*,#27535,.T.);
#36344=ORIENTED_EDGE('',*,*,#27433,.F.);
#36345=ORIENTED_EDGE('',*,*,#27536,.F.);
#36346=ORIENTED_EDGE('',*,*,#27536,.T.);
#36347=ORIENTED_EDGE('',*,*,#27460,.F.);
#36348=ORIENTED_EDGE('',*,*,#27537,.F.);
#36349=ORIENTED_EDGE('',*,*,#27491,.F.);
#36350=ORIENTED_EDGE('',*,*,#27537,.T.);
#36351=ORIENTED_EDGE('',*,*,#27456,.F.);
#36352=ORIENTED_EDGE('',*,*,#27538,.F.);
#36353=ORIENTED_EDGE('',*,*,#27494,.F.);
#36354=ORIENTED_EDGE('',*,*,#27538,.T.);
#36355=ORIENTED_EDGE('',*,*,#27458,.F.);
#36356=ORIENTED_EDGE('',*,*,#27539,.F.);
#36357=ORIENTED_EDGE('',*,*,#27497,.F.);
#36358=ORIENTED_EDGE('',*,*,#27445,.F.);
#36359=ORIENTED_EDGE('',*,*,#27540,.T.);
#36360=ORIENTED_EDGE('',*,*,#27498,.F.);
#36361=ORIENTED_EDGE('',*,*,#27539,.T.);
#36362=ORIENTED_EDGE('',*,*,#27541,.F.);
#36363=ORIENTED_EDGE('',*,*,#27517,.F.);
#36364=ORIENTED_EDGE('',*,*,#27542,.F.);
#36365=ORIENTED_EDGE('',*,*,#27402,.F.);
#36366=ORIENTED_EDGE('',*,*,#27542,.T.);
#36367=ORIENTED_EDGE('',*,*,#27483,.F.);
#36368=ORIENTED_EDGE('',*,*,#27543,.F.);
#36369=ORIENTED_EDGE('',*,*,#27403,.F.);
#36370=ORIENTED_EDGE('',*,*,#27541,.T.);
#36371=ORIENTED_EDGE('',*,*,#27401,.F.);
#36372=ORIENTED_EDGE('',*,*,#27544,.F.);
#36373=ORIENTED_EDGE('',*,*,#27444,.F.);
#36374=ORIENTED_EDGE('',*,*,#27543,.T.);
#36375=ORIENTED_EDGE('',*,*,#27528,.F.);
#36376=ORIENTED_EDGE('',*,*,#27545,.F.);
#36377=ORIENTED_EDGE('',*,*,#27404,.F.);
#36378=ORIENTED_EDGE('',*,*,#27544,.T.);
#36379=ORIENTED_EDGE('',*,*,#27400,.F.);
#36380=ORIENTED_EDGE('',*,*,#27546,.F.);
#36381=ORIENTED_EDGE('',*,*,#27540,.F.);
#36382=ORIENTED_EDGE('',*,*,#27545,.T.);
#36383=ORIENTED_EDGE('',*,*,#27438,.F.);
#36384=ORIENTED_EDGE('',*,*,#27547,.F.);
#36385=ORIENTED_EDGE('',*,*,#27405,.F.);
#36386=ORIENTED_EDGE('',*,*,#27546,.T.);
#36387=ORIENTED_EDGE('',*,*,#27399,.F.);
#36388=ORIENTED_EDGE('',*,*,#27548,.F.);
#36389=ORIENTED_EDGE('',*,*,#27499,.F.);
#36390=ORIENTED_EDGE('',*,*,#27547,.T.);
#36391=ORIENTED_EDGE('',*,*,#27523,.F.);
#36392=ORIENTED_EDGE('',*,*,#27549,.F.);
#36393=ORIENTED_EDGE('',*,*,#27406,.F.);
#36394=ORIENTED_EDGE('',*,*,#27548,.T.);
#36395=ORIENTED_EDGE('',*,*,#27398,.F.);
#36396=ORIENTED_EDGE('',*,*,#27550,.F.);
#36397=ORIENTED_EDGE('',*,*,#27529,.F.);
#36398=ORIENTED_EDGE('',*,*,#27549,.T.);
#36399=ORIENTED_EDGE('',*,*,#27470,.F.);
#36400=ORIENTED_EDGE('',*,*,#27551,.F.);
#36401=ORIENTED_EDGE('',*,*,#27407,.F.);
#36402=ORIENTED_EDGE('',*,*,#27550,.T.);
#36403=ORIENTED_EDGE('',*,*,#27397,.F.);
#36404=ORIENTED_EDGE('',*,*,#27552,.F.);
#36405=ORIENTED_EDGE('',*,*,#27448,.F.);
#36406=ORIENTED_EDGE('',*,*,#27551,.T.);
#36407=ORIENTED_EDGE('',*,*,#27522,.F.);
#36408=ORIENTED_EDGE('',*,*,#27553,.F.);
#36409=ORIENTED_EDGE('',*,*,#27408,.F.);
#36410=ORIENTED_EDGE('',*,*,#27552,.T.);
#36411=ORIENTED_EDGE('',*,*,#27396,.F.);
#36412=ORIENTED_EDGE('',*,*,#27554,.F.);
#36413=ORIENTED_EDGE('',*,*,#27534,.F.);
#36414=ORIENTED_EDGE('',*,*,#27553,.T.);
#36415=ORIENTED_EDGE('',*,*,#27434,.F.);
#36416=ORIENTED_EDGE('',*,*,#27555,.F.);
#36417=ORIENTED_EDGE('',*,*,#27393,.F.);
#36418=ORIENTED_EDGE('',*,*,#27554,.T.);
#36419=ORIENTED_EDGE('',*,*,#27395,.F.);
#36420=ORIENTED_EDGE('',*,*,#27556,.F.);
#36421=ORIENTED_EDGE('',*,*,#27486,.F.);
#36422=ORIENTED_EDGE('',*,*,#27555,.T.);
#36423=ORIENTED_EDGE('',*,*,#27535,.F.);
#36424=ORIENTED_EDGE('',*,*,#27556,.T.);
#36425=ORIENTED_EDGE('',*,*,#27394,.F.);
#42002=TOROIDAL_SURFACE('',#48648,7.,1.);
#42003=TOROIDAL_SURFACE('',#48650,7.,1.);
#42004=TOROIDAL_SURFACE('',#48656,7.,1.);
#42005=TOROIDAL_SURFACE('',#48658,7.,1.);
#42006=TOROIDAL_SURFACE('',#48664,7.,1.);
#42007=TOROIDAL_SURFACE('',#48666,7.,1.);
#42008=TOROIDAL_SURFACE('',#48672,7.,1.);
#42009=TOROIDAL_SURFACE('',#48674,7.,1.);
#42010=TOROIDAL_SURFACE('',#48680,7.00000000000001,1.);
#42011=TOROIDAL_SURFACE('',#48684,7.,1.);
#42012=TOROIDAL_SURFACE('',#48691,2.58578643762686,1.);
#42013=TOROIDAL_SURFACE('',#48695,2.58578643762686,1.);
#42014=TOROIDAL_SURFACE('',#48702,2.58578643762695,1.);
#42015=TOROIDAL_SURFACE('',#48706,2.58578643762694,1.);
#42016=TOROIDAL_SURFACE('',#48713,7.00000000000001,1.);
#42017=TOROIDAL_SURFACE('',#48717,7.,1.);
#42018=TOROIDAL_SURFACE('',#48721,3.,2.);
#42019=TOROIDAL_SURFACE('',#48728,3.,2.);
#42020=TOROIDAL_SURFACE('',#48730,3.,2.);
#42021=TOROIDAL_SURFACE('',#48736,3.,2.);
#42022=TOROIDAL_SURFACE('',#48738,3.,2.);
#42023=TOROIDAL_SURFACE('',#48744,3.,2.);
#42024=TOROIDAL_SURFACE('',#48746,3.,2.);
#42025=TOROIDAL_SURFACE('',#48752,3.,2.);
#43703=ADVANCED_FACE('',(#11123),#8619,.F.);
#43704=ADVANCED_FACE('',(#11124,#721),#3618,.F.);
#43705=ADVANCED_FACE('',(#11125),#3619,.T.);
#43706=ADVANCED_FACE('',(#11126),#3620,.T.);
#43707=ADVANCED_FACE('',(#11127),#3621,.T.);
#43708=ADVANCED_FACE('',(#11128),#3622,.T.);
#43709=ADVANCED_FACE('',(#11129),#3623,.T.);
#43710=ADVANCED_FACE('',(#11130),#3624,.F.);
#43711=ADVANCED_FACE('',(#11131,#722),#3625,.F.);
#43712=ADVANCED_FACE('',(#11132),#3626,.F.);
#43713=ADVANCED_FACE('',(#11133,#723),#3627,.F.);
#43714=ADVANCED_FACE('',(#11134),#3628,.F.);
#43715=ADVANCED_FACE('',(#11135),#8620,.T.);
#43716=ADVANCED_FACE('',(#11136),#8621,.T.);
#43717=ADVANCED_FACE('',(#11137),#8622,.T.);
#43718=ADVANCED_FACE('',(#11138),#8623,.T.);
#43719=ADVANCED_FACE('',(#11139),#8624,.T.);
#43720=ADVANCED_FACE('',(#11140),#8625,.T.);
#43721=ADVANCED_FACE('',(#11141),#3629,.F.);
#43722=ADVANCED_FACE('',(#11142),#78,.T.);
#43723=ADVANCED_FACE('',(#11143),#3630,.F.);
#43724=ADVANCED_FACE('',(#11144),#79,.T.);
#43725=ADVANCED_FACE('',(#11145),#3631,.F.);
#43726=ADVANCED_FACE('',(#11146),#3632,.F.);
#43727=ADVANCED_FACE('',(#11147),#80,.T.);
#43728=ADVANCED_FACE('',(#11148),#3633,.F.);
#43729=ADVANCED_FACE('',(#11149),#81,.T.);
#43730=ADVANCED_FACE('',(#11150),#3634,.F.);
#43731=ADVANCED_FACE('',(#11151),#8626,.T.);
#43732=ADVANCED_FACE('',(#11152),#42002,.T.);
#43733=ADVANCED_FACE('',(#11153),#42003,.T.);
#43734=ADVANCED_FACE('',(#11154),#8627,.T.);
#43735=ADVANCED_FACE('',(#11155),#8628,.T.);
#43736=ADVANCED_FACE('',(#11156),#42004,.T.);
#43737=ADVANCED_FACE('',(#11157),#42005,.T.);
#43738=ADVANCED_FACE('',(#11158),#8629,.T.);
#43739=ADVANCED_FACE('',(#11159),#8630,.T.);
#43740=ADVANCED_FACE('',(#11160),#42006,.T.);
#43741=ADVANCED_FACE('',(#11161),#42007,.T.);
#43742=ADVANCED_FACE('',(#11162),#8631,.T.);
#43743=ADVANCED_FACE('',(#11163),#8632,.T.);
#43744=ADVANCED_FACE('',(#11164),#42008,.T.);
#43745=ADVANCED_FACE('',(#11165),#42009,.T.);
#43746=ADVANCED_FACE('',(#11166),#8633,.T.);
#43747=ADVANCED_FACE('',(#11167),#8634,.T.);
#43748=ADVANCED_FACE('',(#11168),#42010,.T.);
#43749=ADVANCED_FACE('',(#11169),#8635,.T.);
#43750=ADVANCED_FACE('',(#11170),#42011,.T.);
#43751=ADVANCED_FACE('',(#11171),#8636,.T.);
#43752=ADVANCED_FACE('',(#11172),#8637,.T.);
#43753=ADVANCED_FACE('',(#11173),#42012,.T.);
#43754=ADVANCED_FACE('',(#11174),#8638,.T.);
#43755=ADVANCED_FACE('',(#11175),#42013,.T.);
#43756=ADVANCED_FACE('',(#11176),#8639,.T.);
#43757=ADVANCED_FACE('',(#11177),#8640,.T.);
#43758=ADVANCED_FACE('',(#11178),#42014,.T.);
#43759=ADVANCED_FACE('',(#11179),#8641,.T.);
#43760=ADVANCED_FACE('',(#11180),#42015,.T.);
#43761=ADVANCED_FACE('',(#11181),#8642,.T.);
#43762=ADVANCED_FACE('',(#11182),#8643,.T.);
#43763=ADVANCED_FACE('',(#11183),#42016,.T.);
#43764=ADVANCED_FACE('',(#11184),#8644,.T.);
#43765=ADVANCED_FACE('',(#11185),#42017,.T.);
#43766=ADVANCED_FACE('',(#11186),#8645,.T.);
#43767=ADVANCED_FACE('',(#11187),#42018,.F.);
#43768=ADVANCED_FACE('',(#11188),#8646,.F.);
#43769=ADVANCED_FACE('',(#11189),#8647,.F.);
#43770=ADVANCED_FACE('',(#11190),#42019,.F.);
#43771=ADVANCED_FACE('',(#11191),#42020,.F.);
#43772=ADVANCED_FACE('',(#11192),#8648,.F.);
#43773=ADVANCED_FACE('',(#11193),#8649,.F.);
#43774=ADVANCED_FACE('',(#11194),#42021,.F.);
#43775=ADVANCED_FACE('',(#11195),#42022,.F.);
#43776=ADVANCED_FACE('',(#11196),#8650,.F.);
#43777=ADVANCED_FACE('',(#11197),#8651,.F.);
#43778=ADVANCED_FACE('',(#11198),#42023,.F.);
#43779=ADVANCED_FACE('',(#11199),#42024,.F.);
#43780=ADVANCED_FACE('',(#11200),#8652,.F.);
#43781=ADVANCED_FACE('',(#11201),#8653,.F.);
#43782=ADVANCED_FACE('',(#11202),#42025,.F.);
#45456=CLOSED_SHELL('',(#43703,#43704,#43705,#43706,#43707,#43708,#43709,
#43710,#43711,#43712,#43713,#43714,#43715,#43716,#43717,#43718,#43719,#43720,
#43721,#43722,#43723,#43724,#43725,#43726,#43727,#43728,#43729,#43730,#43731,
#43732,#43733,#43734,#43735,#43736,#43737,#43738,#43739,#43740,#43741,#43742,
#43743,#43744,#43745,#43746,#43747,#43748,#43749,#43750,#43751,#43752,#43753,
#43754,#43755,#43756,#43757,#43758,#43759,#43760,#43761,#43762,#43763,#43764,
#43765,#43766,#43767,#43768,#43769,#43770,#43771,#43772,#43773,#43774,#43775,
#43776,#43777,#43778,#43779,#43780,#43781,#43782));
#48574=AXIS2_PLACEMENT_3D('',#96926,#58525,#58526);
#48575=AXIS2_PLACEMENT_3D('',#96927,#58527,#58528);
#48576=AXIS2_PLACEMENT_3D('',#96929,#58529,#58530);
#48577=AXIS2_PLACEMENT_3D('',#96932,#58532,#58533);
#48578=AXIS2_PLACEMENT_3D('',#96933,#58534,#58535);
#48579=AXIS2_PLACEMENT_3D('',#96936,#58536,#58537);
#48580=AXIS2_PLACEMENT_3D('',#96940,#58539,#58540);
#48581=AXIS2_PLACEMENT_3D('',#96944,#58542,#58543);
#48582=AXIS2_PLACEMENT_3D('',#96948,#58545,#58546);
#48583=AXIS2_PLACEMENT_3D('',#96954,#58549,#58550);
#48584=AXIS2_PLACEMENT_3D('',#96958,#58552,#58553);
#48585=AXIS2_PLACEMENT_3D('',#96962,#58555,#58556);
#48586=AXIS2_PLACEMENT_3D('',#96966,#58558,#58559);
#48587=AXIS2_PLACEMENT_3D('',#96970,#58561,#58562);
#48588=AXIS2_PLACEMENT_3D('',#96974,#58564,#58565);
#48589=AXIS2_PLACEMENT_3D('',#96978,#58567,#58568);
#48590=AXIS2_PLACEMENT_3D('',#96981,#58570,#58571);
#48591=AXIS2_PLACEMENT_3D('',#96982,#58572,#58573);
#48592=AXIS2_PLACEMENT_3D('',#96991,#58578,#58579);
#48593=AXIS2_PLACEMENT_3D('',#97000,#58584,#58585);
#48594=AXIS2_PLACEMENT_3D('',#97009,#58590,#58591);
#48595=AXIS2_PLACEMENT_3D('',#97018,#58596,#58597);
#48596=AXIS2_PLACEMENT_3D('',#97021,#58598,#58599);
#48597=AXIS2_PLACEMENT_3D('',#97025,#58601,#58602);
#48598=AXIS2_PLACEMENT_3D('',#97029,#58604,#58605);
#48599=AXIS2_PLACEMENT_3D('',#97033,#58607,#58608);
#48600=AXIS2_PLACEMENT_3D('',#97035,#58610,#58611);
#48601=AXIS2_PLACEMENT_3D('',#97044,#58616,#58617);
#48602=AXIS2_PLACEMENT_3D('',#97053,#58621,#58622);
#48603=AXIS2_PLACEMENT_3D('',#97056,#58624,#58625);
#48604=AXIS2_PLACEMENT_3D('',#97057,#58626,#58627);
#48605=AXIS2_PLACEMENT_3D('',#97066,#58632,#58633);
#48606=AXIS2_PLACEMENT_3D('',#97075,#58637,#58638);
#48607=AXIS2_PLACEMENT_3D('',#97078,#58640,#58641);
#48608=AXIS2_PLACEMENT_3D('',#97079,#58642,#58643);
#48609=AXIS2_PLACEMENT_3D('',#97088,#58648,#58649);
#48610=AXIS2_PLACEMENT_3D('',#97089,#58650,#58651);
#48611=AXIS2_PLACEMENT_3D('',#97090,#58652,#58653);
#48612=AXIS2_PLACEMENT_3D('',#97091,#58654,#58655);
#48613=AXIS2_PLACEMENT_3D('',#97092,#58656,#58657);
#48614=AXIS2_PLACEMENT_3D('',#97093,#58658,#58659);
#48615=AXIS2_PLACEMENT_3D('',#97094,#58660,#58661);
#48616=AXIS2_PLACEMENT_3D('',#97095,#58662,#58663);
#48617=AXIS2_PLACEMENT_3D('',#97096,#58664,#58665);
#48618=AXIS2_PLACEMENT_3D('',#97097,#58666,#58667);
#48619=AXIS2_PLACEMENT_3D('',#97098,#58668,#58669);
#48620=AXIS2_PLACEMENT_3D('',#97099,#58670,#58671);
#48621=AXIS2_PLACEMENT_3D('',#97100,#58672,#58673);
#48622=AXIS2_PLACEMENT_3D('',#97101,#58674,#58675);
#48623=AXIS2_PLACEMENT_3D('',#97102,#58676,#58677);
#48624=AXIS2_PLACEMENT_3D('',#97103,#58678,#58679);
#48625=AXIS2_PLACEMENT_3D('',#97104,#58680,#58681);
#48626=AXIS2_PLACEMENT_3D('',#97105,#58682,#58683);
#48627=AXIS2_PLACEMENT_3D('',#97106,#58684,#58685);
#48628=AXIS2_PLACEMENT_3D('',#97115,#58690,#58691);
#48629=AXIS2_PLACEMENT_3D('',#97119,#58693,#58694);
#48630=AXIS2_PLACEMENT_3D('',#97120,#58695,#58696);
#48631=AXIS2_PLACEMENT_3D('',#97121,#58697,#58698);
#48632=AXIS2_PLACEMENT_3D('',#97127,#58702,#58703);
#48633=AXIS2_PLACEMENT_3D('',#97131,#58705,#58706);
#48634=AXIS2_PLACEMENT_3D('',#97132,#58707,#58708);
#48635=AXIS2_PLACEMENT_3D('',#97133,#58709,#58710);
#48636=AXIS2_PLACEMENT_3D('',#97139,#58714,#58715);
#48637=AXIS2_PLACEMENT_3D('',#97148,#58720,#58721);
#48638=AXIS2_PLACEMENT_3D('',#97152,#58723,#58724);
#48639=AXIS2_PLACEMENT_3D('',#97153,#58725,#58726);
#48640=AXIS2_PLACEMENT_3D('',#97154,#58727,#58728);
#48641=AXIS2_PLACEMENT_3D('',#97160,#58732,#58733);
#48642=AXIS2_PLACEMENT_3D('',#97164,#58735,#58736);
#48643=AXIS2_PLACEMENT_3D('',#97165,#58737,#58738);
#48644=AXIS2_PLACEMENT_3D('',#97166,#58739,#58740);
#48645=AXIS2_PLACEMENT_3D('',#97172,#58744,#58745);
#48646=AXIS2_PLACEMENT_3D('',#97173,#58746,#58747);
#48647=AXIS2_PLACEMENT_3D('',#97174,#58748,#58749);
#48648=AXIS2_PLACEMENT_3D('',#97175,#58750,#58751);
#48649=AXIS2_PLACEMENT_3D('',#97176,#58752,#58753);
#48650=AXIS2_PLACEMENT_3D('',#97177,#58754,#58755);
#48651=AXIS2_PLACEMENT_3D('',#97178,#58756,#58757);
#48652=AXIS2_PLACEMENT_3D('',#97179,#58758,#58759);
#48653=AXIS2_PLACEMENT_3D('',#97180,#58760,#58761);
#48654=AXIS2_PLACEMENT_3D('',#97181,#58762,#58763);
#48655=AXIS2_PLACEMENT_3D('',#97182,#58764,#58765);
#48656=AXIS2_PLACEMENT_3D('',#97183,#58766,#58767);
#48657=AXIS2_PLACEMENT_3D('',#97184,#58768,#58769);
#48658=AXIS2_PLACEMENT_3D('',#97185,#58770,#58771);
#48659=AXIS2_PLACEMENT_3D('',#97186,#58772,#58773);
#48660=AXIS2_PLACEMENT_3D('',#97187,#58774,#58775);
#48661=AXIS2_PLACEMENT_3D('',#97188,#58776,#58777);
#48662=AXIS2_PLACEMENT_3D('',#97189,#58778,#58779);
#48663=AXIS2_PLACEMENT_3D('',#97190,#58780,#58781);
#48664=AXIS2_PLACEMENT_3D('',#97191,#58782,#58783);
#48665=AXIS2_PLACEMENT_3D('',#97192,#58784,#58785);
#48666=AXIS2_PLACEMENT_3D('',#97193,#58786,#58787);
#48667=AXIS2_PLACEMENT_3D('',#97194,#58788,#58789);
#48668=AXIS2_PLACEMENT_3D('',#97195,#58790,#58791);
#48669=AXIS2_PLACEMENT_3D('',#97196,#58792,#58793);
#48670=AXIS2_PLACEMENT_3D('',#97197,#58794,#58795);
#48671=AXIS2_PLACEMENT_3D('',#97198,#58796,#58797);
#48672=AXIS2_PLACEMENT_3D('',#97199,#58798,#58799);
#48673=AXIS2_PLACEMENT_3D('',#97200,#58800,#58801);
#48674=AXIS2_PLACEMENT_3D('',#97201,#58802,#58803);
#48675=AXIS2_PLACEMENT_3D('',#97202,#58804,#58805);
#48676=AXIS2_PLACEMENT_3D('',#97203,#58806,#58807);
#48677=AXIS2_PLACEMENT_3D('',#97204,#58808,#58809);
#48678=AXIS2_PLACEMENT_3D('',#97205,#58810,#58811);
#48679=AXIS2_PLACEMENT_3D('',#97206,#58812,#58813);
#48680=AXIS2_PLACEMENT_3D('',#97207,#58814,#58815);
#48681=AXIS2_PLACEMENT_3D('',#97208,#58816,#58817);
#48682=AXIS2_PLACEMENT_3D('',#97209,#58818,#58819);
#48683=AXIS2_PLACEMENT_3D('',#97210,#58820,#58821);
#48684=AXIS2_PLACEMENT_3D('',#97211,#58822,#58823);
#48685=AXIS2_PLACEMENT_3D('',#97212,#58824,#58825);
#48686=AXIS2_PLACEMENT_3D('',#97213,#58826,#58827);
#48687=AXIS2_PLACEMENT_3D('',#97214,#58828,#58829);
#48688=AXIS2_PLACEMENT_3D('',#97215,#58830,#58831);
#48689=AXIS2_PLACEMENT_3D('',#97216,#58832,#58833);
#48690=AXIS2_PLACEMENT_3D('',#97217,#58834,#58835);
#48691=AXIS2_PLACEMENT_3D('',#97218,#58836,#58837);
#48692=AXIS2_PLACEMENT_3D('',#97219,#58838,#58839);
#48693=AXIS2_PLACEMENT_3D('',#97220,#58840,#58841);
#48694=AXIS2_PLACEMENT_3D('',#97221,#58842,#58843);
#48695=AXIS2_PLACEMENT_3D('',#97222,#58844,#58845);
#48696=AXIS2_PLACEMENT_3D('',#97223,#58846,#58847);
#48697=AXIS2_PLACEMENT_3D('',#97224,#58848,#58849);
#48698=AXIS2_PLACEMENT_3D('',#97225,#58850,#58851);
#48699=AXIS2_PLACEMENT_3D('',#97226,#58852,#58853);
#48700=AXIS2_PLACEMENT_3D('',#97227,#58854,#58855);
#48701=AXIS2_PLACEMENT_3D('',#97228,#58856,#58857);
#48702=AXIS2_PLACEMENT_3D('',#97229,#58858,#58859);
#48703=AXIS2_PLACEMENT_3D('',#97230,#58860,#58861);
#48704=AXIS2_PLACEMENT_3D('',#97231,#58862,#58863);
#48705=AXIS2_PLACEMENT_3D('',#97232,#58864,#58865);
#48706=AXIS2_PLACEMENT_3D('',#97233,#58866,#58867);
#48707=AXIS2_PLACEMENT_3D('',#97234,#58868,#58869);
#48708=AXIS2_PLACEMENT_3D('',#97235,#58870,#58871);
#48709=AXIS2_PLACEMENT_3D('',#97236,#58872,#58873);
#48710=AXIS2_PLACEMENT_3D('',#97237,#58874,#58875);
#48711=AXIS2_PLACEMENT_3D('',#97238,#58876,#58877);
#48712=AXIS2_PLACEMENT_3D('',#97239,#58878,#58879);
#48713=AXIS2_PLACEMENT_3D('',#97240,#58880,#58881);
#48714=AXIS2_PLACEMENT_3D('',#97241,#58882,#58883);
#48715=AXIS2_PLACEMENT_3D('',#97242,#58884,#58885);
#48716=AXIS2_PLACEMENT_3D('',#97243,#58886,#58887);
#48717=AXIS2_PLACEMENT_3D('',#97244,#58888,#58889);
#48718=AXIS2_PLACEMENT_3D('',#97245,#58890,#58891);
#48719=AXIS2_PLACEMENT_3D('',#97246,#58892,#58893);
#48720=AXIS2_PLACEMENT_3D('',#97247,#58894,#58895);
#48721=AXIS2_PLACEMENT_3D('',#97248,#58896,#58897);
#48722=AXIS2_PLACEMENT_3D('',#97249,#58898,#58899);
#48723=AXIS2_PLACEMENT_3D('',#97250,#58900,#58901);
#48724=AXIS2_PLACEMENT_3D('',#97251,#58902,#58903);
#48725=AXIS2_PLACEMENT_3D('',#97252,#58904,#58905);
#48726=AXIS2_PLACEMENT_3D('',#97253,#58906,#58907);
#48727=AXIS2_PLACEMENT_3D('',#97254,#58908,#58909);
#48728=AXIS2_PLACEMENT_3D('',#97255,#58910,#58911);
#48729=AXIS2_PLACEMENT_3D('',#97256,#58912,#58913);
#48730=AXIS2_PLACEMENT_3D('',#97257,#58914,#58915);
#48731=AXIS2_PLACEMENT_3D('',#97258,#58916,#58917);
#48732=AXIS2_PLACEMENT_3D('',#97259,#58918,#58919);
#48733=AXIS2_PLACEMENT_3D('',#97260,#58920,#58921);
#48734=AXIS2_PLACEMENT_3D('',#97261,#58922,#58923);
#48735=AXIS2_PLACEMENT_3D('',#97262,#58924,#58925);
#48736=AXIS2_PLACEMENT_3D('',#97263,#58926,#58927);
#48737=AXIS2_PLACEMENT_3D('',#97264,#58928,#58929);
#48738=AXIS2_PLACEMENT_3D('',#97265,#58930,#58931);
#48739=AXIS2_PLACEMENT_3D('',#97266,#58932,#58933);
#48740=AXIS2_PLACEMENT_3D('',#97267,#58934,#58935);
#48741=AXIS2_PLACEMENT_3D('',#97268,#58936,#58937);
#48742=AXIS2_PLACEMENT_3D('',#97269,#58938,#58939);
#48743=AXIS2_PLACEMENT_3D('',#97270,#58940,#58941);
#48744=AXIS2_PLACEMENT_3D('',#97271,#58942,#58943);
#48745=AXIS2_PLACEMENT_3D('',#97272,#58944,#58945);
#48746=AXIS2_PLACEMENT_3D('',#97273,#58946,#58947);
#48747=AXIS2_PLACEMENT_3D('',#97274,#58948,#58949);
#48748=AXIS2_PLACEMENT_3D('',#97275,#58950,#58951);
#48749=AXIS2_PLACEMENT_3D('',#97276,#58952,#58953);
#48750=AXIS2_PLACEMENT_3D('',#97277,#58954,#58955);
#48751=AXIS2_PLACEMENT_3D('',#97278,#58956,#58957);
#48752=AXIS2_PLACEMENT_3D('',#97279,#58958,#58959);
#58525=DIRECTION('axis',(0.,0.,1.));
#58526=DIRECTION('refdir',(1.,0.,0.));
#58527=DIRECTION('center_axis',(0.,1.,0.));
#58528=DIRECTION('ref_axis',(0.,0.,1.));
#58529=DIRECTION('center_axis',(0.,1.,0.));
#58530=DIRECTION('ref_axis',(0.,0.,1.));
#58531=DIRECTION('',(0.,1.,0.));
#58532=DIRECTION('center_axis',(0.,1.,0.));
#58533=DIRECTION('ref_axis',(0.,0.,1.));
#58534=DIRECTION('center_axis',(0.,0.,-1.));
#58535=DIRECTION('ref_axis',(-1.,0.,0.));
#58536=DIRECTION('center_axis',(0.,0.,1.));
#58537=DIRECTION('ref_axis',(-1.,0.,0.));
#58538=DIRECTION('',(-1.,0.,0.));
#58539=DIRECTION('center_axis',(0.,0.,1.));
#58540=DIRECTION('ref_axis',(-1.,0.,0.));
#58541=DIRECTION('',(0.,-1.,0.));
#58542=DIRECTION('center_axis',(0.,0.,1.));
#58543=DIRECTION('ref_axis',(-1.,0.,0.));
#58544=DIRECTION('',(1.,0.,0.));
#58545=DIRECTION('center_axis',(0.,0.,1.));
#58546=DIRECTION('ref_axis',(-1.,0.,0.));
#58547=DIRECTION('',(0.,1.,0.));
#58548=DIRECTION('',(0.,1.,0.));
#58549=DIRECTION('center_axis',(0.,0.,-1.));
#58550=DIRECTION('ref_axis',(-1.,0.,0.));
#58551=DIRECTION('',(0.70710678118655,0.707106781186544,0.));
#58552=DIRECTION('center_axis',(0.,0.,-1.));
#58553=DIRECTION('ref_axis',(-1.,0.,0.));
#58554=DIRECTION('',(1.,0.,0.));
#58555=DIRECTION('center_axis',(0.,0.,-1.));
#58556=DIRECTION('ref_axis',(-1.,0.,0.));
#58557=DIRECTION('',(0.707106781186551,-0.707106781186544,0.));
#58558=DIRECTION('center_axis',(0.,0.,-1.));
#58559=DIRECTION('ref_axis',(-1.,0.,0.));
#58560=DIRECTION('',(0.,-1.,0.));
#58561=DIRECTION('center_axis',(0.,0.,-1.));
#58562=DIRECTION('ref_axis',(-1.,0.,0.));
#58563=DIRECTION('',(-0.707106781186548,-0.707106781186546,0.));
#58564=DIRECTION('center_axis',(0.,0.,-1.));
#58565=DIRECTION('ref_axis',(-1.,0.,0.));
#58566=DIRECTION('',(-1.,0.,0.));
#58567=DIRECTION('center_axis',(0.,0.,-1.));
#58568=DIRECTION('ref_axis',(-1.,0.,0.));
#58569=DIRECTION('',(-0.707106781186548,0.707106781186546,0.));
#58570=DIRECTION('center_axis',(0.,0.,-1.));
#58571=DIRECTION('ref_axis',(-1.,0.,0.));
#58572=DIRECTION('center_axis',(-1.,0.,0.));
#58573=DIRECTION('ref_axis',(0.,0.,1.));
#58574=DIRECTION('',(0.,0.,-1.));
#58575=DIRECTION('',(0.,-1.,0.));
#58576=DIRECTION('',(0.,0.,1.));
#58577=DIRECTION('',(0.,1.,0.));
#58578=DIRECTION('center_axis',(0.,-1.,0.));
#58579=DIRECTION('ref_axis',(0.,0.,-1.));
#58580=DIRECTION('',(0.,0.,-1.));
#58581=DIRECTION('',(1.,0.,0.));
#58582=DIRECTION('',(0.,0.,1.));
#58583=DIRECTION('',(-1.,0.,0.));
#58584=DIRECTION('center_axis',(1.,0.,0.));
#58585=DIRECTION('ref_axis',(0.,0.,-1.));
#58586=DIRECTION('',(0.,0.,-1.));
#58587=DIRECTION('',(0.,1.,0.));
#58588=DIRECTION('',(0.,0.,1.));
#58589=DIRECTION('',(0.,-1.,0.));
#58590=DIRECTION('center_axis',(0.,1.,0.));
#58591=DIRECTION('ref_axis',(0.,0.,1.));
#58592=DIRECTION('',(0.,0.,-1.));
#58593=DIRECTION('',(-1.,0.,0.));
#58594=DIRECTION('',(0.,0.,1.));
#58595=DIRECTION('',(1.,0.,0.));
#58596=DIRECTION('center_axis',(0.,0.,-1.));
#58597=DIRECTION('ref_axis',(-1.,0.,0.));
#58598=DIRECTION('center_axis',(0.,0.,-1.));
#58599=DIRECTION('ref_axis',(-1.,0.,0.));
#58600=DIRECTION('',(0.,1.,0.));
#58601=DIRECTION('center_axis',(0.,0.,-1.));
#58602=DIRECTION('ref_axis',(-1.,0.,0.));
#58603=DIRECTION('',(1.,0.,0.));
#58604=DIRECTION('center_axis',(0.,0.,-1.));
#58605=DIRECTION('ref_axis',(-1.,0.,0.));
#58606=DIRECTION('',(0.,-1.,0.));
#58607=DIRECTION('center_axis',(0.,0.,-1.));
#58608=DIRECTION('ref_axis',(-1.,0.,0.));
#58609=DIRECTION('',(-1.,0.,0.));
#58610=DIRECTION('center_axis',(1.,0.,0.));
#58611=DIRECTION('ref_axis',(0.,0.,-1.));
#58612=DIRECTION('',(0.,0.,-1.));
#58613=DIRECTION('',(0.,-1.,0.));
#58614=DIRECTION('',(0.,0.,1.));
#58615=DIRECTION('',(0.,1.,0.));
#58616=DIRECTION('center_axis',(0.,1.,0.));
#58617=DIRECTION('ref_axis',(0.,0.,1.));
#58618=DIRECTION('',(0.,0.,-1.));
#58619=DIRECTION('',(1.,0.,0.));
#58620=DIRECTION('',(0.,0.,1.));
#58621=DIRECTION('center_axis',(0.,-1.,0.));
#58622=DIRECTION('ref_axis',(0.,0.,1.));
#58623=DIRECTION('',(-1.,0.,0.));
#58624=DIRECTION('center_axis',(0.,-1.,0.));
#58625=DIRECTION('ref_axis',(0.,0.,1.));
#58626=DIRECTION('center_axis',(-1.,0.,0.));
#58627=DIRECTION('ref_axis',(0.,0.,1.));
#58628=DIRECTION('',(0.,0.,-1.));
#58629=DIRECTION('',(0.,1.,0.));
#58630=DIRECTION('',(0.,0.,1.));
#58631=DIRECTION('',(0.,-1.,0.));
#58632=DIRECTION('center_axis',(0.,-1.,0.));
#58633=DIRECTION('ref_axis',(0.,0.,-1.));
#58634=DIRECTION('',(0.,0.,-1.));
#58635=DIRECTION('',(-1.,0.,0.));
#58636=DIRECTION('',(0.,0.,1.));
#58637=DIRECTION('center_axis',(0.,1.,0.));
#58638=DIRECTION('ref_axis',(0.,0.,-1.));
#58639=DIRECTION('',(1.,0.,0.));
#58640=DIRECTION('center_axis',(0.,1.,0.));
#58641=DIRECTION('ref_axis',(0.,0.,-1.));
#58642=DIRECTION('center_axis',(0.,0.,-1.));
#58643=DIRECTION('ref_axis',(-1.,0.,0.));
#58644=DIRECTION('',(0.,-1.,0.));
#58645=DIRECTION('',(1.,0.,0.));
#58646=DIRECTION('',(0.,1.,0.));
#58647=DIRECTION('',(-1.,0.,0.));
#58648=DIRECTION('center_axis',(0.,1.,0.));
#58649=DIRECTION('ref_axis',(0.,0.,1.));
#58650=DIRECTION('center_axis',(0.,1.,0.));
#58651=DIRECTION('ref_axis',(0.,0.,-1.));
#58652=DIRECTION('center_axis',(0.,-1.,0.));
#58653=DIRECTION('ref_axis',(0.,0.,1.));
#58654=DIRECTION('center_axis',(0.,-1.,0.));
#58655=DIRECTION('ref_axis',(0.,0.,-1.));
#58656=DIRECTION('center_axis',(0.,1.,0.));
#58657=DIRECTION('ref_axis',(0.,0.,-1.));
#58658=DIRECTION('center_axis',(0.,-1.,0.));
#58659=DIRECTION('ref_axis',(0.,0.,1.));
#58660=DIRECTION('center_axis',(0.,0.,-1.));
#58661=DIRECTION('ref_axis',(-1.,0.,0.));
#58662=DIRECTION('center_axis',(0.,0.,1.));
#58663=DIRECTION('ref_axis',(-1.,0.,0.));
#58664=DIRECTION('center_axis',(0.,0.,-1.));
#58665=DIRECTION('ref_axis',(-1.,0.,0.));
#58666=DIRECTION('center_axis',(0.,0.,-1.));
#58667=DIRECTION('ref_axis',(-1.,0.,0.));
#58668=DIRECTION('center_axis',(0.,0.,1.));
#58669=DIRECTION('ref_axis',(-1.,0.,0.));
#58670=DIRECTION('center_axis',(0.,0.,-1.));
#58671=DIRECTION('ref_axis',(-1.,0.,0.));
#58672=DIRECTION('center_axis',(0.,0.,-1.));
#58673=DIRECTION('ref_axis',(-1.,0.,0.));
#58674=DIRECTION('center_axis',(0.,0.,1.));
#58675=DIRECTION('ref_axis',(-1.,0.,0.));
#58676=DIRECTION('center_axis',(0.,0.,-1.));
#58677=DIRECTION('ref_axis',(-1.,0.,0.));
#58678=DIRECTION('center_axis',(0.,0.,-1.));
#58679=DIRECTION('ref_axis',(-1.,0.,0.));
#58680=DIRECTION('center_axis',(0.,0.,1.));
#58681=DIRECTION('ref_axis',(-1.,0.,0.));
#58682=DIRECTION('center_axis',(0.,0.,-1.));
#58683=DIRECTION('ref_axis',(-1.,0.,0.));
#58684=DIRECTION('center_axis',(0.707106781186547,0.707106781186549,0.));
#58685=DIRECTION('ref_axis',(0.,0.,-1.));
#58686=DIRECTION('',(0.,0.,-1.));
#58687=DIRECTION('',(0.707106781186549,-0.707106781186546,0.));
#58688=DIRECTION('',(0.,0.,1.));
#58689=DIRECTION('',(0.707106781186548,-0.707106781186546,0.));
#58690=DIRECTION('center_axis',(0.,1.,0.));
#58691=DIRECTION('ref_axis',(0.,0.,1.));
#58692=DIRECTION('',(0.,-0.707106781186546,-0.707106781186548));
#58693=DIRECTION('center_axis',(0.,-1.,0.));
#58694=DIRECTION('ref_axis',(0.,0.,-1.));
#58695=DIRECTION('center_axis',(0.,1.,0.));
#58696=DIRECTION('ref_axis',(0.,0.,1.));
#58697=DIRECTION('center_axis',(0.,0.707106781186549,-0.707106781186547));
#58698=DIRECTION('ref_axis',(1.,0.,0.));
#58699=DIRECTION('',(0.,-0.707106781186546,-0.707106781186548));
#58700=DIRECTION('',(-1.,0.,0.));
#58701=DIRECTION('',(1.,0.,0.));
#58702=DIRECTION('center_axis',(0.,1.,0.));
#58703=DIRECTION('ref_axis',(0.,0.,1.));
#58704=DIRECTION('',(-0.707106781186549,-0.707106781186546,0.));
#58705=DIRECTION('center_axis',(0.,-1.,0.));
#58706=DIRECTION('ref_axis',(0.,0.,-1.));
#58707=DIRECTION('center_axis',(0.,1.,0.));
#58708=DIRECTION('ref_axis',(0.,0.,1.));
#58709=DIRECTION('center_axis',(-0.707106781186547,0.707106781186549,0.));
#58710=DIRECTION('ref_axis',(0.,0.,-1.));
#58711=DIRECTION('',(0.,0.,-1.));
#58712=DIRECTION('',(0.707106781186549,0.707106781186547,0.));
#58713=DIRECTION('',(0.,0.,1.));
#58714=DIRECTION('center_axis',(0.707106781186545,-0.707106781186551,0.));
#58715=DIRECTION('ref_axis',(0.,0.,-1.));
#58716=DIRECTION('',(0.,0.,-1.));
#58717=DIRECTION('',(-0.70710678118655,-0.707106781186544,0.));
#58718=DIRECTION('',(0.,0.,1.));
#58719=DIRECTION('',(-0.70710678118655,-0.707106781186544,0.));
#58720=DIRECTION('center_axis',(0.,-1.,0.));
#58721=DIRECTION('ref_axis',(0.,0.,-1.));
#58722=DIRECTION('',(0.,-0.707106781186544,0.70710678118655));
#58723=DIRECTION('center_axis',(0.,-1.,0.));
#58724=DIRECTION('ref_axis',(0.,0.,-1.));
#58725=DIRECTION('center_axis',(0.,1.,0.));
#58726=DIRECTION('ref_axis',(0.,0.,1.));
#58727=DIRECTION('center_axis',(0.,-0.707106781186551,-0.707106781186545));
#58728=DIRECTION('ref_axis',(-1.,0.,0.));
#58729=DIRECTION('',(0.,-0.707106781186544,0.70710678118655));
#58730=DIRECTION('',(-1.,0.,0.));
#58731=DIRECTION('',(1.,0.,0.));
#58732=DIRECTION('center_axis',(0.,-1.,0.));
#58733=DIRECTION('ref_axis',(0.,0.,-1.));
#58734=DIRECTION('',(0.707106781186551,-0.707106781186544,0.));
#58735=DIRECTION('center_axis',(0.,-1.,0.));
#58736=DIRECTION('ref_axis',(0.,0.,-1.));
#58737=DIRECTION('center_axis',(0.,1.,0.));
#58738=DIRECTION('ref_axis',(0.,0.,1.));
#58739=DIRECTION('center_axis',(-0.707106781186544,-0.707106781186551,0.));
#58740=DIRECTION('ref_axis',(0.,0.,-1.));
#58741=DIRECTION('',(0.,0.,-1.));
#58742=DIRECTION('',(-0.707106781186551,0.707106781186544,0.));
#58743=DIRECTION('',(0.,0.,1.));
#58744=DIRECTION('center_axis',(0.,-1.,0.));
#58745=DIRECTION('ref_axis',(0.,0.,-1.));
#58746=DIRECTION('center_axis',(0.,1.,0.));
#58747=DIRECTION('ref_axis',(0.,0.,1.));
#58748=DIRECTION('center_axis',(0.,-1.,0.));
#58749=DIRECTION('ref_axis',(0.,0.,-1.));
#58750=DIRECTION('center_axis',(0.,0.,-1.));
#58751=DIRECTION('ref_axis',(-1.,0.,0.));
#58752=DIRECTION('center_axis',(-1.,0.,0.));
#58753=DIRECTION('ref_axis',(0.,0.,1.));
#58754=DIRECTION('center_axis',(0.,0.,-1.));
#58755=DIRECTION('ref_axis',(-1.,0.,0.));
#58756=DIRECTION('center_axis',(-1.,0.,0.));
#58757=DIRECTION('ref_axis',(0.,0.,1.));
#58758=DIRECTION('center_axis',(-1.,0.,0.));
#58759=DIRECTION('ref_axis',(0.,0.,1.));
#58760=DIRECTION('center_axis',(-1.,0.,0.));
#58761=DIRECTION('ref_axis',(0.,0.,1.));
#58762=DIRECTION('center_axis',(1.,0.,0.));
#58763=DIRECTION('ref_axis',(0.,0.,-1.));
#58764=DIRECTION('center_axis',(-1.,0.,0.));
#58765=DIRECTION('ref_axis',(0.,0.,1.));
#58766=DIRECTION('center_axis',(0.,0.,-1.));
#58767=DIRECTION('ref_axis',(-1.,0.,0.));
#58768=DIRECTION('center_axis',(0.,1.,0.));
#58769=DIRECTION('ref_axis',(0.,0.,1.));
#58770=DIRECTION('center_axis',(0.,0.,-1.));
#58771=DIRECTION('ref_axis',(-1.,0.,0.));
#58772=DIRECTION('center_axis',(0.,-1.,0.));
#58773=DIRECTION('ref_axis',(0.,0.,-1.));
#58774=DIRECTION('center_axis',(0.,1.,0.));
#58775=DIRECTION('ref_axis',(0.,0.,1.));
#58776=DIRECTION('center_axis',(1.,0.,0.));
#58777=DIRECTION('ref_axis',(0.,0.,-1.));
#58778=DIRECTION('center_axis',(1.,0.,0.));
#58779=DIRECTION('ref_axis',(0.,0.,-1.));
#58780=DIRECTION('center_axis',(-1.,0.,0.));
#58781=DIRECTION('ref_axis',(0.,0.,1.));
#58782=DIRECTION('center_axis',(0.,0.,-1.));
#58783=DIRECTION('ref_axis',(-1.,0.,0.));
#58784=DIRECTION('center_axis',(0.,1.,0.));
#58785=DIRECTION('ref_axis',(0.,0.,1.));
#58786=DIRECTION('center_axis',(0.,0.,-1.));
#58787=DIRECTION('ref_axis',(-1.,0.,0.));
#58788=DIRECTION('center_axis',(0.,1.,0.));
#58789=DIRECTION('ref_axis',(0.,0.,1.));
#58790=DIRECTION('center_axis',(0.,-1.,0.));
#58791=DIRECTION('ref_axis',(0.,0.,-1.));
#58792=DIRECTION('center_axis',(0.,1.,0.));
#58793=DIRECTION('ref_axis',(0.,0.,1.));
#58794=DIRECTION('center_axis',(0.,1.,0.));
#58795=DIRECTION('ref_axis',(0.,0.,1.));
#58796=DIRECTION('center_axis',(0.,1.,0.));
#58797=DIRECTION('ref_axis',(0.,0.,1.));
#58798=DIRECTION('center_axis',(0.,0.,-1.));
#58799=DIRECTION('ref_axis',(-1.,0.,0.));
#58800=DIRECTION('center_axis',(1.,0.,0.));
#58801=DIRECTION('ref_axis',(0.,0.,-1.));
#58802=DIRECTION('center_axis',(0.,0.,-1.));
#58803=DIRECTION('ref_axis',(-1.,0.,0.));
#58804=DIRECTION('center_axis',(-1.,0.,0.));
#58805=DIRECTION('ref_axis',(0.,0.,1.));
#58806=DIRECTION('center_axis',(-1.,0.,0.));
#58807=DIRECTION('ref_axis',(0.,0.,1.));
#58808=DIRECTION('center_axis',(0.,0.,-1.));
#58809=DIRECTION('ref_axis',(-1.,0.,0.));
#58810=DIRECTION('center_axis',(0.,0.,1.));
#58811=DIRECTION('ref_axis',(-1.,-1.11022302462516E-13,0.));
#58812=DIRECTION('center_axis',(0.,0.,1.));
#58813=DIRECTION('ref_axis',(1.,0.,0.));
#58814=DIRECTION('center_axis',(0.,-1.,0.));
#58815=DIRECTION('ref_axis',(0.,0.,-1.));
#58816=DIRECTION('center_axis',(-1.,0.,0.));
#58817=DIRECTION('ref_axis',(0.,0.,1.));
#58818=DIRECTION('center_axis',(1.,0.,0.));
#58819=DIRECTION('ref_axis',(0.,0.,-1.));
#58820=DIRECTION('center_axis',(-1.,0.,0.));
#58821=DIRECTION('ref_axis',(0.,0.,1.));
#58822=DIRECTION('center_axis',(0.,-1.,0.));
#58823=DIRECTION('ref_axis',(0.,0.,-1.));
#58824=DIRECTION('center_axis',(0.,0.,-1.));
#58825=DIRECTION('ref_axis',(-1.,0.,0.));
#58826=DIRECTION('center_axis',(0.,0.,1.));
#58827=DIRECTION('ref_axis',(1.,0.,0.));
#58828=DIRECTION('center_axis',(0.,0.,1.));
#58829=DIRECTION('ref_axis',(-1.,0.,0.));
#58830=DIRECTION('center_axis',(0.,0.,-1.));
#58831=DIRECTION('ref_axis',(-1.,0.,0.));
#58832=DIRECTION('center_axis',(0.,0.,1.));
#58833=DIRECTION('ref_axis',(-1.,0.,0.));
#58834=DIRECTION('center_axis',(0.,0.,1.));
#58835=DIRECTION('ref_axis',(1.,0.,0.));
#58836=DIRECTION('center_axis',(0.,1.,0.));
#58837=DIRECTION('ref_axis',(0.,0.,1.));
#58838=DIRECTION('center_axis',(1.,0.,0.));
#58839=DIRECTION('ref_axis',(0.,0.,-1.));
#58840=DIRECTION('center_axis',(-1.,0.,0.));
#58841=DIRECTION('ref_axis',(0.,0.,1.));
#58842=DIRECTION('center_axis',(1.,0.,0.));
#58843=DIRECTION('ref_axis',(0.,0.,-1.));
#58844=DIRECTION('center_axis',(0.,1.,0.));
#58845=DIRECTION('ref_axis',(0.,0.,1.));
#58846=DIRECTION('center_axis',(0.,0.,-1.));
#58847=DIRECTION('ref_axis',(-1.,0.,0.));
#58848=DIRECTION('center_axis',(0.,0.,1.));
#58849=DIRECTION('ref_axis',(1.,0.,0.));
#58850=DIRECTION('center_axis',(0.,0.,1.));
#58851=DIRECTION('ref_axis',(-1.,0.,0.));
#58852=DIRECTION('center_axis',(0.,0.,-1.));
#58853=DIRECTION('ref_axis',(-1.,0.,0.));
#58854=DIRECTION('center_axis',(0.,0.,1.));
#58855=DIRECTION('ref_axis',(-1.,1.11022302462516E-13,0.));
#58856=DIRECTION('center_axis',(0.,0.,1.));
#58857=DIRECTION('ref_axis',(1.,0.,0.));
#58858=DIRECTION('center_axis',(0.,-1.,0.));
#58859=DIRECTION('ref_axis',(0.,0.,-1.));
#58860=DIRECTION('center_axis',(-1.,0.,0.));
#58861=DIRECTION('ref_axis',(0.,0.,1.));
#58862=DIRECTION('center_axis',(1.,0.,0.));
#58863=DIRECTION('ref_axis',(0.,0.,-1.));
#58864=DIRECTION('center_axis',(-1.,0.,0.));
#58865=DIRECTION('ref_axis',(0.,0.,1.));
#58866=DIRECTION('center_axis',(0.,-1.,0.));
#58867=DIRECTION('ref_axis',(0.,0.,-1.));
#58868=DIRECTION('center_axis',(0.,0.,-1.));
#58869=DIRECTION('ref_axis',(-1.,0.,0.));
#58870=DIRECTION('center_axis',(0.,0.,1.));
#58871=DIRECTION('ref_axis',(1.,0.,0.));
#58872=DIRECTION('center_axis',(0.,0.,1.));
#58873=DIRECTION('ref_axis',(-1.,1.11022302462516E-13,0.));
#58874=DIRECTION('center_axis',(0.,0.,-1.));
#58875=DIRECTION('ref_axis',(-1.,0.,0.));
#58876=DIRECTION('center_axis',(0.,0.,1.));
#58877=DIRECTION('ref_axis',(-1.,-2.22044604925031E-13,0.));
#58878=DIRECTION('center_axis',(0.,0.,1.));
#58879=DIRECTION('ref_axis',(1.,0.,0.));
#58880=DIRECTION('center_axis',(0.,1.,0.));
#58881=DIRECTION('ref_axis',(0.,0.,1.));
#58882=DIRECTION('center_axis',(1.,0.,0.));
#58883=DIRECTION('ref_axis',(0.,0.,-1.));
#58884=DIRECTION('center_axis',(-1.,0.,0.));
#58885=DIRECTION('ref_axis',(0.,0.,1.));
#58886=DIRECTION('center_axis',(1.,0.,0.));
#58887=DIRECTION('ref_axis',(0.,0.,-1.));
#58888=DIRECTION('center_axis',(0.,1.,0.));
#58889=DIRECTION('ref_axis',(0.,0.,1.));
#58890=DIRECTION('center_axis',(0.,0.,-1.));
#58891=DIRECTION('ref_axis',(-1.,0.,0.));
#58892=DIRECTION('center_axis',(0.,0.,1.));
#58893=DIRECTION('ref_axis',(1.,0.,0.));
#58894=DIRECTION('center_axis',(0.,0.,1.));
#58895=DIRECTION('ref_axis',(-1.,-1.11022302462516E-13,0.));
#58896=DIRECTION('center_axis',(0.,0.,-1.));
#58897=DIRECTION('ref_axis',(-1.,0.,0.));
#58898=DIRECTION('center_axis',(0.,-1.,0.));
#58899=DIRECTION('ref_axis',(0.,0.,-1.));
#58900=DIRECTION('center_axis',(0.707106781186535,0.70710678118656,0.));
#58901=DIRECTION('ref_axis',(-0.70710678118656,0.707106781186535,0.));
#58902=DIRECTION('center_axis',(0.707106781186549,0.707106781186547,0.));
#58903=DIRECTION('ref_axis',(-0.707106781186547,0.707106781186549,0.));
#58904=DIRECTION('center_axis',(0.707106781186561,0.707106781186534,0.));
#58905=DIRECTION('ref_axis',(-0.707106781186534,0.707106781186561,0.));
#58906=DIRECTION('center_axis',(0.,-1.,0.));
#58907=DIRECTION('ref_axis',(0.,0.,-1.));
#58908=DIRECTION('center_axis',(0.,-1.,0.));
#58909=DIRECTION('ref_axis',(0.,0.,-1.));
#58910=DIRECTION('center_axis',(0.,0.,-1.));
#58911=DIRECTION('ref_axis',(-1.,0.,0.));
#58912=DIRECTION('center_axis',(1.,0.,0.));
#58913=DIRECTION('ref_axis',(0.,0.,-1.));
#58914=DIRECTION('center_axis',(0.,0.,-1.));
#58915=DIRECTION('ref_axis',(-1.,0.,0.));
#58916=DIRECTION('center_axis',(0.707106781186567,-0.707106781186528,0.));
#58917=DIRECTION('ref_axis',(0.707106781186528,0.707106781186567,0.));
#58918=DIRECTION('center_axis',(-1.,0.,0.));
#58919=DIRECTION('ref_axis',(0.,0.,1.));
#58920=DIRECTION('center_axis',(1.,0.,0.));
#58921=DIRECTION('ref_axis',(0.,0.,-1.));
#58922=DIRECTION('center_axis',(-0.707106781186551,0.707106781186544,0.));
#58923=DIRECTION('ref_axis',(-0.707106781186544,-0.707106781186551,0.));
#58924=DIRECTION('center_axis',(0.707106781186561,-0.707106781186534,1.59462515335074E-14));
#58925=DIRECTION('ref_axis',(0.707106781186534,0.707106781186561,1.36377391314472E-28));
#58926=DIRECTION('center_axis',(0.,0.,-1.));
#58927=DIRECTION('ref_axis',(-1.,0.,0.));
#58928=DIRECTION('center_axis',(0.707106781186565,-0.70710678118653,0.));
#58929=DIRECTION('ref_axis',(0.70710678118653,0.707106781186565,0.));
#58930=DIRECTION('center_axis',(0.,0.,-1.));
#58931=DIRECTION('ref_axis',(-1.,0.,0.));
#58932=DIRECTION('center_axis',(1.,0.,0.));
#58933=DIRECTION('ref_axis',(0.,0.,-1.));
#58934=DIRECTION('center_axis',(0.707106781186549,-0.707106781186547,0.));
#58935=DIRECTION('ref_axis',(0.707106781186547,0.707106781186549,0.));
#58936=DIRECTION('center_axis',(0.70710678118656,-0.707106781186535,0.));
#58937=DIRECTION('ref_axis',(0.707106781186535,0.70710678118656,0.));
#58938=DIRECTION('center_axis',(1.,0.,0.));
#58939=DIRECTION('ref_axis',(0.,0.,-1.));
#58940=DIRECTION('center_axis',(1.,0.,0.));
#58941=DIRECTION('ref_axis',(0.,0.,-1.));
#58942=DIRECTION('center_axis',(0.,0.,-1.));
#58943=DIRECTION('ref_axis',(-1.,0.,0.));
#58944=DIRECTION('center_axis',(0.,-1.,0.));
#58945=DIRECTION('ref_axis',(0.,0.,-1.));
#58946=DIRECTION('center_axis',(0.,0.,-1.));
#58947=DIRECTION('ref_axis',(-1.,0.,0.));
#58948=DIRECTION('center_axis',(0.707106781186568,0.707106781186527,0.));
#58949=DIRECTION('ref_axis',(-0.707106781186527,0.707106781186568,0.));
#58950=DIRECTION('center_axis',(0.,1.,0.));
#58951=DIRECTION('ref_axis',(0.,0.,1.));
#58952=DIRECTION('center_axis',(0.,-1.,0.));
#58953=DIRECTION('ref_axis',(0.,0.,-1.));
#58954=DIRECTION('center_axis',(-0.70710678118655,-0.707106781186545,0.));
#58955=DIRECTION('ref_axis',(0.707106781186545,-0.707106781186551,0.));
#58956=DIRECTION('center_axis',(0.707106781186561,0.707106781186534,2.45326946669344E-15));
#58957=DIRECTION('ref_axis',(-0.707106781186534,0.707106781186561,-1.81613594474679E-29));
#58958=DIRECTION('center_axis',(0.,0.,-1.));
#58959=DIRECTION('ref_axis',(-1.,0.,0.));
#96926=CARTESIAN_POINT('',(0.,0.,0.));
#96927=CARTESIAN_POINT('Origin',(0.,799.524274233158,64.2994740882088));
#96928=CARTESIAN_POINT('',(-1.46957615897682E-15,819.591294394281,52.2994740882088));
#96929=CARTESIAN_POINT('Origin',(0.,819.591294394281,64.2994740882088));
#96930=CARTESIAN_POINT('',(-1.46957615897682E-15,842.524274233158,52.2994740882088));
#96931=CARTESIAN_POINT('',(-1.46957615897682E-15,799.524274233158,52.2994740882088));
#96932=CARTESIAN_POINT('Origin',(0.,842.524274233158,64.2994740882088));
#96933=CARTESIAN_POINT('Origin',(0.,0.,48.));
#96934=CARTESIAN_POINT('',(44.0626743494,846.77801102117,48.));
#96935=CARTESIAN_POINT('',(37.0626743494,853.77801102117,48.));
#96936=CARTESIAN_POINT('Origin',(37.0626743494,846.77801102117,48.));
#96937=CARTESIAN_POINT('',(-37.0626743494,853.77801102117,48.));
#96938=CARTESIAN_POINT('',(-37.0626743494,853.77801102117,48.));
#96939=CARTESIAN_POINT('',(-44.0626743494,846.77801102117,48.));
#96940=CARTESIAN_POINT('Origin',(-37.0626743494,846.77801102117,48.));
#96941=CARTESIAN_POINT('',(-44.0626743494,816.144821069057,48.));
#96942=CARTESIAN_POINT('',(-44.0626743494,816.144821069057,48.));
#96943=CARTESIAN_POINT('',(-37.0626743494,809.144821069057,48.));
#96944=CARTESIAN_POINT('Origin',(-37.0626743494,816.144821069057,48.));
#96945=CARTESIAN_POINT('',(37.0626743494,809.144821069057,48.));
#96946=CARTESIAN_POINT('',(37.0626743494,809.144821069057,48.));
#96947=CARTESIAN_POINT('',(44.0626743494,816.144821069057,48.));
#96948=CARTESIAN_POINT('Origin',(37.0626743494,816.144821069057,48.));
#96949=CARTESIAN_POINT('',(44.0626743494,846.77801102117,48.));
#96950=CARTESIAN_POINT('',(-34.9669957384604,825.005507956654,48.));
#96951=CARTESIAN_POINT('',(-34.9669957384604,837.110060670785,48.));
#96952=CARTESIAN_POINT('',(-34.9669957384604,837.110060670785,48.));
#96953=CARTESIAN_POINT('',(-34.08831608202,839.231381014344,48.));
#96954=CARTESIAN_POINT('Origin',(-31.9669957384604,837.110060670785,48.));
#96955=CARTESIAN_POINT('',(-29.674102519647,843.645594576717,48.));
#96956=CARTESIAN_POINT('',(-436.659848548182,436.659848548186,48.));
#96957=CARTESIAN_POINT('',(-27.5527821760873,844.524274233158,48.));
#96958=CARTESIAN_POINT('Origin',(-27.5527821760873,841.524274233158,48.));
#96959=CARTESIAN_POINT('',(27.5527821760873,844.524274233158,48.));
#96960=CARTESIAN_POINT('',(27.5527821760873,844.524274233158,48.));
#96961=CARTESIAN_POINT('',(29.674102519647,843.645594576717,48.));
#96962=CARTESIAN_POINT('Origin',(27.5527821760873,841.524274233158,48.));
#96963=CARTESIAN_POINT('',(34.0883160820201,839.231381014345,48.));
#96964=CARTESIAN_POINT('',(436.659848548182,436.659848548186,48.));
#96965=CARTESIAN_POINT('',(34.9669957384604,837.110060670785,48.));
#96966=CARTESIAN_POINT('Origin',(31.9669957384604,837.110060670785,48.));
#96967=CARTESIAN_POINT('',(34.9669957384604,825.005507956654,48.));
#96968=CARTESIAN_POINT('',(34.9669957384604,825.005507956654,48.));
#96969=CARTESIAN_POINT('',(34.08831608202,822.884187613094,48.));
#96970=CARTESIAN_POINT('Origin',(31.9669957384604,825.005507956654,48.));
#96971=CARTESIAN_POINT('',(29.6741025196469,818.469974050721,48.));
#96972=CARTESIAN_POINT('',(-394.397935765537,394.397935765538,48.));
#96973=CARTESIAN_POINT('',(27.5527821760872,817.591294394281,48.));
#96974=CARTESIAN_POINT('Origin',(27.5527821760872,820.591294394281,48.));
#96975=CARTESIAN_POINT('',(-27.5527821760872,817.591294394281,48.));
#96976=CARTESIAN_POINT('',(-27.5527821760872,817.591294394281,48.));
#96977=CARTESIAN_POINT('',(-29.6741025196469,818.469974050721,48.));
#96978=CARTESIAN_POINT('Origin',(-27.5527821760872,820.591294394281,48.));
#96979=CARTESIAN_POINT('',(-34.08831608202,822.884187613094,48.));
#96980=CARTESIAN_POINT('',(394.397935765537,394.397935765538,48.));
#96981=CARTESIAN_POINT('Origin',(-31.9669957384604,825.005507956654,48.));
#96982=CARTESIAN_POINT('Origin',(-45.0626743494,854.77801102117,48.));
#96983=CARTESIAN_POINT('',(-45.0626743494,846.77801102117,47.));
#96984=CARTESIAN_POINT('',(-45.0626743494,846.77801102117,41.));
#96985=CARTESIAN_POINT('',(-45.0626743494,846.77801102117,48.));
#96986=CARTESIAN_POINT('',(-45.0626743494,816.144821069057,41.));
#96987=CARTESIAN_POINT('',(-45.0626743494,854.77801102117,41.));
#96988=CARTESIAN_POINT('',(-45.0626743494,816.144821069057,47.));
#96989=CARTESIAN_POINT('',(-45.0626743494,816.144821069057,48.));
#96990=CARTESIAN_POINT('',(-45.0626743494,846.77801102117,47.));
#96991=CARTESIAN_POINT('Origin',(45.0626743494,808.144821069057,48.));
#96992=CARTESIAN_POINT('',(-37.0626743494,808.144821069057,47.));
#96993=CARTESIAN_POINT('',(-37.0626743494,808.144821069057,41.));
#96994=CARTESIAN_POINT('',(-37.0626743494,808.144821069057,48.));
#96995=CARTESIAN_POINT('',(37.0626743494,808.144821069057,41.));
#96996=CARTESIAN_POINT('',(45.0626743494,808.144821069057,41.));
#96997=CARTESIAN_POINT('',(37.0626743494,808.144821069057,47.));
#96998=CARTESIAN_POINT('',(37.0626743494,808.144821069057,48.));
#96999=CARTESIAN_POINT('',(-37.0626743494,808.144821069057,47.));
#97000=CARTESIAN_POINT('Origin',(45.0626743494,854.77801102117,48.));
#97001=CARTESIAN_POINT('',(45.0626743494,816.144821069057,47.));
#97002=CARTESIAN_POINT('',(45.0626743494,816.144821069057,41.));
#97003=CARTESIAN_POINT('',(45.0626743494,816.144821069057,48.));
#97004=CARTESIAN_POINT('',(45.0626743494,846.77801102117,41.));
#97005=CARTESIAN_POINT('',(45.0626743494,854.77801102117,41.));
#97006=CARTESIAN_POINT('',(45.0626743494,846.77801102117,47.));
#97007=CARTESIAN_POINT('',(45.0626743494,846.77801102117,48.));
#97008=CARTESIAN_POINT('',(45.0626743494,816.144821069057,47.));
#97009=CARTESIAN_POINT('Origin',(45.0626743494,854.77801102117,48.));
#97010=CARTESIAN_POINT('',(37.0626743494,854.77801102117,47.));
#97011=CARTESIAN_POINT('',(37.0626743494,854.77801102117,41.));
#97012=CARTESIAN_POINT('',(37.0626743494,854.77801102117,48.));
#97013=CARTESIAN_POINT('',(-37.0626743494,854.77801102117,41.));
#97014=CARTESIAN_POINT('',(45.0626743494,854.77801102117,41.));
#97015=CARTESIAN_POINT('',(-37.0626743494,854.77801102117,47.));
#97016=CARTESIAN_POINT('',(-37.0626743494,854.77801102117,48.));
#97017=CARTESIAN_POINT('',(37.0626743494,854.77801102117,47.));
#97018=CARTESIAN_POINT('Origin',(0.,0.,40.));
#97019=CARTESIAN_POINT('',(-37.0626743494,809.144821069057,40.));
#97020=CARTESIAN_POINT('',(-44.0626743494,816.144821069057,40.));
#97021=CARTESIAN_POINT('Origin',(-37.0626743494,816.144821069057,40.));
#97022=CARTESIAN_POINT('',(-44.0626743494,846.77801102117,40.));
#97023=CARTESIAN_POINT('',(-44.0626743494,0.,40.));
#97024=CARTESIAN_POINT('',(-37.0626743494,853.77801102117,40.));
#97025=CARTESIAN_POINT('Origin',(-37.0626743494,846.77801102117,40.));
#97026=CARTESIAN_POINT('',(37.0626743494,853.77801102117,40.));
#97027=CARTESIAN_POINT('',(0.,853.77801102117,40.));
#97028=CARTESIAN_POINT('',(44.0626743494,846.77801102117,40.));
#97029=CARTESIAN_POINT('Origin',(37.0626743494,846.77801102117,40.));
#97030=CARTESIAN_POINT('',(44.0626743494,816.144821069057,40.));
#97031=CARTESIAN_POINT('',(44.0626743494,0.,40.));
#97032=CARTESIAN_POINT('',(37.0626743494,809.144821069057,40.));
#97033=CARTESIAN_POINT('Origin',(37.0626743494,816.144821069057,40.));
#97034=CARTESIAN_POINT('',(0.,809.144821069057,40.));
#97035=CARTESIAN_POINT('Origin',(-32.9669957384604,842.524274233158,91.));
#97036=CARTESIAN_POINT('',(-32.9669957384604,837.110060670785,83.));
#97037=CARTESIAN_POINT('',(-32.9669957384604,837.110060670785,50.));
#97038=CARTESIAN_POINT('',(-32.9669957384604,837.110060670785,48.));
#97039=CARTESIAN_POINT('',(-32.9669957384604,825.005507956654,50.));
#97040=CARTESIAN_POINT('',(-32.9669957384604,825.005507956654,50.));
#97041=CARTESIAN_POINT('',(-32.9669957384604,825.005507956654,83.));
#97042=CARTESIAN_POINT('',(-32.9669957384604,825.005507956654,83.));
#97043=CARTESIAN_POINT('',(-32.9669957384604,842.524274233158,83.));
#97044=CARTESIAN_POINT('Origin',(32.9669957384604,819.591294394281,91.));
#97045=CARTESIAN_POINT('',(-27.5527821760872,819.591294394281,83.));
#97046=CARTESIAN_POINT('',(-27.5527821760872,819.591294394281,50.));
#97047=CARTESIAN_POINT('',(-27.5527821760872,819.591294394281,48.));
#97048=CARTESIAN_POINT('',(27.5527821760872,819.591294394281,50.));
#97049=CARTESIAN_POINT('',(27.5527821760872,819.591294394281,50.));
#97050=CARTESIAN_POINT('',(27.5527821760872,819.591294394281,83.));
#97051=CARTESIAN_POINT('',(27.5527821760872,819.591294394281,83.));
#97052=CARTESIAN_POINT('',(24.9669957384604,819.591294394281,85.5857864376269));
#97053=CARTESIAN_POINT('Origin',(24.9669957384604,819.591294394281,83.));
#97054=CARTESIAN_POINT('',(-24.9669957384604,819.591294394281,85.5857864376269));
#97055=CARTESIAN_POINT('',(-24.9669957384604,819.591294394281,85.5857864376269));
#97056=CARTESIAN_POINT('Origin',(-24.9669957384604,819.591294394281,83.));
#97057=CARTESIAN_POINT('Origin',(32.9669957384604,842.524274233158,91.));
#97058=CARTESIAN_POINT('',(32.9669957384604,825.005507956654,83.));
#97059=CARTESIAN_POINT('',(32.9669957384604,825.005507956654,50.));
#97060=CARTESIAN_POINT('',(32.9669957384604,825.005507956654,48.));
#97061=CARTESIAN_POINT('',(32.9669957384604,837.110060670785,50.));
#97062=CARTESIAN_POINT('',(32.9669957384604,837.110060670785,50.));
#97063=CARTESIAN_POINT('',(32.9669957384604,837.110060670785,83.));
#97064=CARTESIAN_POINT('',(32.9669957384604,837.110060670785,83.));
#97065=CARTESIAN_POINT('',(32.9669957384604,842.524274233158,83.));
#97066=CARTESIAN_POINT('Origin',(32.9669957384604,842.524274233158,91.));
#97067=CARTESIAN_POINT('',(27.5527821760873,842.524274233158,83.));
#97068=CARTESIAN_POINT('',(27.5527821760873,842.524274233158,50.));
#97069=CARTESIAN_POINT('',(27.5527821760873,842.524274233158,48.));
#97070=CARTESIAN_POINT('',(-27.5527821760873,842.524274233158,50.));
#97071=CARTESIAN_POINT('',(-27.5527821760873,842.524274233158,50.));
#97072=CARTESIAN_POINT('',(-27.5527821760873,842.524274233158,83.));
#97073=CARTESIAN_POINT('',(-27.5527821760873,842.524274233158,83.));
#97074=CARTESIAN_POINT('',(-24.9669957384604,842.524274233158,85.585786437627));
#97075=CARTESIAN_POINT('Origin',(-24.9669957384604,842.524274233158,83.));
#97076=CARTESIAN_POINT('',(24.9669957384604,842.524274233158,85.585786437627));
#97077=CARTESIAN_POINT('',(24.9669957384604,842.524274233158,85.585786437627));
#97078=CARTESIAN_POINT('Origin',(24.9669957384604,842.524274233158,83.));
#97079=CARTESIAN_POINT('Origin',(0.,0.,91.));
#97080=CARTESIAN_POINT('',(-24.9669957384604,837.110060670785,91.));
#97081=CARTESIAN_POINT('',(-24.9669957384604,825.005507956654,91.));
#97082=CARTESIAN_POINT('',(-24.9669957384604,0.,91.));
#97083=CARTESIAN_POINT('',(24.9669957384604,825.005507956654,91.));
#97084=CARTESIAN_POINT('',(24.9669957384604,825.005507956654,91.));
#97085=CARTESIAN_POINT('',(24.9669957384604,837.110060670785,91.));
#97086=CARTESIAN_POINT('',(24.9669957384604,0.,91.));
#97087=CARTESIAN_POINT('',(-24.9669957384604,837.110060670785,91.));
#97088=CARTESIAN_POINT('Origin',(24.9669957384604,0.,83.));
#97089=CARTESIAN_POINT('Origin',(24.9669957384604,825.005507956654,83.));
#97090=CARTESIAN_POINT('Origin',(24.9669957384604,837.110060670785,83.));
#97091=CARTESIAN_POINT('Origin',(-24.9669957384604,0.,83.));
#97092=CARTESIAN_POINT('Origin',(-24.9669957384604,825.005507956654,83.));
#97093=CARTESIAN_POINT('Origin',(-24.9669957384604,837.110060670785,83.));
#97094=CARTESIAN_POINT('Origin',(37.0626743494,846.77801102117,48.));
#97095=CARTESIAN_POINT('Origin',(37.0626743494,846.77801102117,41.));
#97096=CARTESIAN_POINT('Origin',(37.0626743494,846.77801102117,47.));
#97097=CARTESIAN_POINT('Origin',(37.0626743494,816.144821069057,48.));
#97098=CARTESIAN_POINT('Origin',(37.0626743494,816.144821069057,41.));
#97099=CARTESIAN_POINT('Origin',(37.0626743494,816.144821069057,47.));
#97100=CARTESIAN_POINT('Origin',(-37.0626743494,816.144821069057,48.));
#97101=CARTESIAN_POINT('Origin',(-37.0626743494,816.144821069057,41.));
#97102=CARTESIAN_POINT('Origin',(-37.0626743494,816.144821069057,47.));
#97103=CARTESIAN_POINT('Origin',(-37.0626743494,846.77801102117,48.));
#97104=CARTESIAN_POINT('Origin',(-37.0626743494,846.77801102117,41.));
#97105=CARTESIAN_POINT('Origin',(-37.0626743494,846.77801102117,47.));
#97106=CARTESIAN_POINT('Origin',(-27.9669957384604,819.591294394281,91.));
#97107=CARTESIAN_POINT('',(-32.6741025196469,824.298401175467,83.));
#97108=CARTESIAN_POINT('',(-32.6741025196469,824.298401175467,50.));
#97109=CARTESIAN_POINT('',(-32.6741025196469,824.298401175467,48.));
#97110=CARTESIAN_POINT('',(-28.2598889572738,819.884187613094,50.));
#97111=CARTESIAN_POINT('',(-27.9669957384604,819.591294394281,50.));
#97112=CARTESIAN_POINT('',(-28.2598889572738,819.884187613094,83.));
#97113=CARTESIAN_POINT('',(-28.2598889572738,819.884187613094,83.));
#97114=CARTESIAN_POINT('',(-32.9669957384604,824.591294394281,83.));
#97115=CARTESIAN_POINT('Origin',(-24.9669957384604,819.591294394281,83.));
#97116=CARTESIAN_POINT('',(-24.9669957384604,824.298401175467,90.7071067811866));
#97117=CARTESIAN_POINT('',(-24.9669957384604,819.884187613094,86.2928932188134));
#97118=CARTESIAN_POINT('',(-24.9669957384604,824.591294394281,91.));
#97119=CARTESIAN_POINT('Origin',(-24.9669957384604,824.298401175467,83.));
#97120=CARTESIAN_POINT('Origin',(-24.9669957384604,819.884187613094,83.));
#97121=CARTESIAN_POINT('Origin',(0.,824.591294394281,91.));
#97122=CARTESIAN_POINT('',(24.9669957384604,824.298401175467,90.7071067811866));
#97123=CARTESIAN_POINT('',(24.9669957384604,819.884187613094,86.2928932188134));
#97124=CARTESIAN_POINT('',(24.9669957384604,824.591294394281,91.));
#97125=CARTESIAN_POINT('',(-24.9669957384604,824.298401175467,90.7071067811866));
#97126=CARTESIAN_POINT('',(24.9669957384604,819.884187613094,86.2928932188134));
#97127=CARTESIAN_POINT('Origin',(24.9669957384604,819.591294394281,83.));
#97128=CARTESIAN_POINT('',(32.6741025196469,824.298401175467,83.));
#97129=CARTESIAN_POINT('',(28.2598889572738,819.884187613094,83.));
#97130=CARTESIAN_POINT('',(32.9669957384604,824.591294394281,83.));
#97131=CARTESIAN_POINT('Origin',(24.9669957384604,824.298401175467,83.));
#97132=CARTESIAN_POINT('Origin',(24.9669957384604,819.884187613094,83.));
#97133=CARTESIAN_POINT('Origin',(32.9669957384604,824.591294394281,91.));
#97134=CARTESIAN_POINT('',(28.2598889572738,819.884187613094,50.));
#97135=CARTESIAN_POINT('',(28.2598889572738,819.884187613094,48.));
#97136=CARTESIAN_POINT('',(32.6741025196469,824.298401175467,50.));
#97137=CARTESIAN_POINT('',(32.9669957384604,824.591294394281,50.));
#97138=CARTESIAN_POINT('',(32.6741025196469,824.298401175467,83.));
#97139=CARTESIAN_POINT('Origin',(-32.9669957384604,837.524274233158,91.));
#97140=CARTESIAN_POINT('',(-28.2598889572739,842.231381014344,83.));
#97141=CARTESIAN_POINT('',(-28.2598889572739,842.231381014344,50.));
#97142=CARTESIAN_POINT('',(-28.2598889572739,842.231381014344,48.));
#97143=CARTESIAN_POINT('',(-32.6741025196469,837.817167451971,50.));
#97144=CARTESIAN_POINT('',(-32.9669957384604,837.524274233158,50.));
#97145=CARTESIAN_POINT('',(-32.6741025196469,837.817167451971,83.));
#97146=CARTESIAN_POINT('',(-32.6741025196469,837.817167451971,83.));
#97147=CARTESIAN_POINT('',(-27.9669957384604,842.524274233158,83.));
#97148=CARTESIAN_POINT('Origin',(-24.9669957384604,842.524274233158,83.));
#97149=CARTESIAN_POINT('',(-24.9669957384604,842.231381014344,86.2928932188135));
#97150=CARTESIAN_POINT('',(-24.9669957384604,837.817167451971,90.7071067811866));
#97151=CARTESIAN_POINT('',(-24.9669957384604,842.524274233158,86.0000000000001));
#97152=CARTESIAN_POINT('Origin',(-24.9669957384604,842.231381014344,83.));
#97153=CARTESIAN_POINT('Origin',(-24.9669957384604,837.817167451971,83.));
#97154=CARTESIAN_POINT('Origin',(0.,837.524274233158,91.));
#97155=CARTESIAN_POINT('',(24.9669957384604,842.231381014344,86.2928932188135));
#97156=CARTESIAN_POINT('',(24.9669957384604,837.817167451971,90.7071067811866));
#97157=CARTESIAN_POINT('',(24.9669957384604,842.524274233158,86.0000000000001));
#97158=CARTESIAN_POINT('',(-24.9669957384604,842.231381014344,86.2928932188135));
#97159=CARTESIAN_POINT('',(24.9669957384604,837.817167451971,90.7071067811866));
#97160=CARTESIAN_POINT('Origin',(24.9669957384604,842.524274233158,83.));
#97161=CARTESIAN_POINT('',(28.2598889572739,842.231381014344,83.));
#97162=CARTESIAN_POINT('',(32.6741025196469,837.817167451971,83.));
#97163=CARTESIAN_POINT('',(27.9669957384604,842.524274233158,83.));
#97164=CARTESIAN_POINT('Origin',(24.9669957384604,842.231381014344,83.));
#97165=CARTESIAN_POINT('Origin',(24.9669957384604,837.817167451971,83.));
#97166=CARTESIAN_POINT('Origin',(27.9669957384604,842.524274233158,91.));
#97167=CARTESIAN_POINT('',(32.6741025196469,837.817167451971,50.));
#97168=CARTESIAN_POINT('',(32.6741025196469,837.817167451971,48.));
#97169=CARTESIAN_POINT('',(28.2598889572739,842.231381014344,50.));
#97170=CARTESIAN_POINT('',(27.9669957384604,842.524274233158,50.));
#97171=CARTESIAN_POINT('',(28.2598889572739,842.231381014344,83.));
#97172=CARTESIAN_POINT('Origin',(44.0626743494,0.,41.));
#97173=CARTESIAN_POINT('Origin',(44.0626743494,846.77801102117,41.));
#97174=CARTESIAN_POINT('Origin',(44.0626743494,816.144821069057,41.));
#97175=CARTESIAN_POINT('Origin',(37.0626743494,816.144821069057,41.));
#97176=CARTESIAN_POINT('Origin',(37.0626743494,809.144821069057,41.));
#97177=CARTESIAN_POINT('Origin',(37.0626743494,846.77801102117,41.));
#97178=CARTESIAN_POINT('Origin',(37.0626743494,853.77801102117,41.));
#97179=CARTESIAN_POINT('Origin',(0.,809.144821069057,41.));
#97180=CARTESIAN_POINT('Origin',(-37.0626743494,809.144821069057,41.));
#97181=CARTESIAN_POINT('Origin',(0.,853.77801102117,41.));
#97182=CARTESIAN_POINT('Origin',(-37.0626743494,853.77801102117,41.));
#97183=CARTESIAN_POINT('Origin',(-37.0626743494,816.144821069057,41.));
#97184=CARTESIAN_POINT('Origin',(-44.0626743494,816.144821069057,41.));
#97185=CARTESIAN_POINT('Origin',(-37.0626743494,846.77801102117,41.));
#97186=CARTESIAN_POINT('Origin',(-44.0626743494,846.77801102117,41.));
#97187=CARTESIAN_POINT('Origin',(-44.0626743494,0.,41.));
#97188=CARTESIAN_POINT('Origin',(45.0626743494,809.144821069057,47.));
#97189=CARTESIAN_POINT('Origin',(37.0626743494,809.144821069057,47.));
#97190=CARTESIAN_POINT('Origin',(-37.0626743494,809.144821069057,47.));
#97191=CARTESIAN_POINT('Origin',(-37.0626743494,816.144821069057,47.));
#97192=CARTESIAN_POINT('Origin',(-44.0626743494,816.144821069057,47.));
#97193=CARTESIAN_POINT('Origin',(37.0626743494,816.144821069057,47.));
#97194=CARTESIAN_POINT('Origin',(44.0626743494,816.144821069057,47.));
#97195=CARTESIAN_POINT('Origin',(-44.0626743494,854.77801102117,47.));
#97196=CARTESIAN_POINT('Origin',(-44.0626743494,846.77801102117,47.));
#97197=CARTESIAN_POINT('Origin',(44.0626743494,854.77801102117,47.));
#97198=CARTESIAN_POINT('Origin',(44.0626743494,846.77801102117,47.));
#97199=CARTESIAN_POINT('Origin',(-37.0626743494,846.77801102117,47.));
#97200=CARTESIAN_POINT('Origin',(-37.0626743494,853.77801102117,47.));
#97201=CARTESIAN_POINT('Origin',(37.0626743494,846.77801102117,47.));
#97202=CARTESIAN_POINT('Origin',(37.0626743494,853.77801102117,47.));
#97203=CARTESIAN_POINT('Origin',(45.0626743494,853.77801102117,47.));
#97204=CARTESIAN_POINT('Origin',(31.9669957384604,825.005507956654,91.));
#97205=CARTESIAN_POINT('Origin',(31.9669957384604,825.005507956654,50.));
#97206=CARTESIAN_POINT('Origin',(31.9669957384604,825.005507956654,83.));
#97207=CARTESIAN_POINT('Origin',(24.9669957384604,825.005507956654,83.));
#97208=CARTESIAN_POINT('Origin',(24.9669957384604,825.005507956654,90.0000000000001));
#97209=CARTESIAN_POINT('Origin',(0.,825.005507956654,90.));
#97210=CARTESIAN_POINT('Origin',(-24.9669957384604,825.005507956654,90.0000000000001));
#97211=CARTESIAN_POINT('Origin',(-24.9669957384604,825.005507956654,83.));
#97212=CARTESIAN_POINT('Origin',(-31.9669957384604,825.005507956654,83.));
#97213=CARTESIAN_POINT('Origin',(-31.9669957384604,825.005507956654,91.));
#97214=CARTESIAN_POINT('Origin',(-31.9669957384604,825.005507956654,50.));
#97215=CARTESIAN_POINT('Origin',(-27.5527821760872,820.591294394281,91.));
#97216=CARTESIAN_POINT('Origin',(-27.5527821760872,820.591294394281,50.));
#97217=CARTESIAN_POINT('Origin',(-27.5527821760873,820.591294394281,83.));
#97218=CARTESIAN_POINT('Origin',(-24.9669957384604,820.591294394281,83.));
#97219=CARTESIAN_POINT('Origin',(-24.9669957384604,820.591294394281,85.5857864376269));
#97220=CARTESIAN_POINT('Origin',(32.9669957384604,820.591294394281,85.5857864376269));
#97221=CARTESIAN_POINT('Origin',(24.9669957384604,820.591294394281,85.5857864376269));
#97222=CARTESIAN_POINT('Origin',(24.9669957384604,820.591294394281,83.));
#97223=CARTESIAN_POINT('Origin',(27.5527821760872,820.591294394281,83.));
#97224=CARTESIAN_POINT('Origin',(27.5527821760872,820.591294394281,91.));
#97225=CARTESIAN_POINT('Origin',(27.5527821760872,820.591294394281,50.));
#97226=CARTESIAN_POINT('Origin',(27.5527821760873,841.524274233158,91.));
#97227=CARTESIAN_POINT('Origin',(27.5527821760873,841.524274233158,50.));
#97228=CARTESIAN_POINT('Origin',(27.5527821760873,841.524274233158,83.));
#97229=CARTESIAN_POINT('Origin',(24.9669957384604,841.524274233158,83.));
#97230=CARTESIAN_POINT('Origin',(24.9669957384604,841.524274233158,85.585786437627));
#97231=CARTESIAN_POINT('Origin',(32.9669957384604,841.524274233158,85.585786437627));
#97232=CARTESIAN_POINT('Origin',(-24.9669957384604,841.524274233158,85.585786437627));
#97233=CARTESIAN_POINT('Origin',(-24.9669957384604,841.524274233158,83.));
#97234=CARTESIAN_POINT('Origin',(-27.5527821760873,841.524274233158,83.));
#97235=CARTESIAN_POINT('Origin',(-27.5527821760873,841.524274233158,91.));
#97236=CARTESIAN_POINT('Origin',(-27.5527821760873,841.524274233158,50.));
#97237=CARTESIAN_POINT('Origin',(-31.9669957384604,837.110060670785,91.));
#97238=CARTESIAN_POINT('Origin',(-31.9669957384604,837.110060670785,50.));
#97239=CARTESIAN_POINT('Origin',(-31.9669957384604,837.110060670785,83.));
#97240=CARTESIAN_POINT('Origin',(-24.9669957384604,837.110060670785,83.));
#97241=CARTESIAN_POINT('Origin',(-24.9669957384604,837.110060670785,90.0000000000001));
#97242=CARTESIAN_POINT('Origin',(0.,837.110060670785,90.));
#97243=CARTESIAN_POINT('Origin',(24.9669957384604,837.110060670785,90.0000000000001));
#97244=CARTESIAN_POINT('Origin',(24.9669957384604,837.110060670785,83.));
#97245=CARTESIAN_POINT('Origin',(31.9669957384604,837.110060670785,83.));
#97246=CARTESIAN_POINT('Origin',(31.9669957384604,837.110060670785,91.));
#97247=CARTESIAN_POINT('Origin',(31.9669957384604,837.110060670785,50.));
#97248=CARTESIAN_POINT('Origin',(31.9669957384604,825.005507956654,50.));
#97249=CARTESIAN_POINT('Origin',(34.9669957384604,825.005507956654,50.));
#97250=CARTESIAN_POINT('Origin',(34.08831608202,822.884187613094,50.));
#97251=CARTESIAN_POINT('Origin',(-394.397935765537,394.397935765538,50.));
#97252=CARTESIAN_POINT('Origin',(29.6741025196469,818.469974050721,50.));
#97253=CARTESIAN_POINT('Origin',(34.9669957384604,842.524274233158,50.));
#97254=CARTESIAN_POINT('Origin',(34.9669957384604,837.110060670785,50.));
#97255=CARTESIAN_POINT('Origin',(27.5527821760872,820.591294394281,50.));
#97256=CARTESIAN_POINT('Origin',(27.5527821760872,817.591294394281,50.));
#97257=CARTESIAN_POINT('Origin',(31.9669957384604,837.110060670785,50.));
#97258=CARTESIAN_POINT('Origin',(34.08831608202,839.231381014344,50.));
#97259=CARTESIAN_POINT('Origin',(32.9669957384604,817.591294394281,50.));
#97260=CARTESIAN_POINT('Origin',(-27.5527821760872,817.591294394281,50.));
#97261=CARTESIAN_POINT('Origin',(436.659848548182,436.659848548186,50.));
#97262=CARTESIAN_POINT('Origin',(29.674102519647,843.645594576717,50.));
#97263=CARTESIAN_POINT('Origin',(-27.5527821760872,820.591294394281,50.));
#97264=CARTESIAN_POINT('Origin',(-29.6741025196469,818.469974050721,50.));
#97265=CARTESIAN_POINT('Origin',(27.5527821760873,841.524274233158,50.));
#97266=CARTESIAN_POINT('Origin',(27.5527821760873,844.524274233158,50.));
#97267=CARTESIAN_POINT('Origin',(394.397935765537,394.397935765538,50.));
#97268=CARTESIAN_POINT('Origin',(-34.08831608202,822.884187613094,50.));
#97269=CARTESIAN_POINT('Origin',(32.9669957384604,844.524274233158,50.));
#97270=CARTESIAN_POINT('Origin',(-27.5527821760873,844.524274233158,50.));
#97271=CARTESIAN_POINT('Origin',(-31.9669957384604,825.005507956654,50.));
#97272=CARTESIAN_POINT('Origin',(-34.9669957384604,825.005507956654,50.));
#97273=CARTESIAN_POINT('Origin',(-27.5527821760873,841.524274233158,50.));
#97274=CARTESIAN_POINT('Origin',(-29.6741025196469,843.645594576717,50.));
#97275=CARTESIAN_POINT('Origin',(-34.9669957384604,842.524274233158,50.));
#97276=CARTESIAN_POINT('Origin',(-34.9669957384604,837.110060670785,50.));
#97277=CARTESIAN_POINT('Origin',(-436.659848548182,436.659848548186,50.));
#97278=CARTESIAN_POINT('Origin',(-34.08831608202,839.231381014344,50.));
#97279=CARTESIAN_POINT('Origin',(-31.9669957384604,837.110060670785,50.));
#130896=UNCERTAINTY_MEASURE_WITH_UNIT(LENGTH_MEASURE(0.01),#130911,
'DISTANCE_ACCURACY_VALUE',
'Maximum model space distance between geometric entities at asserted c
onnectivities');
#130900=UNCERTAINTY_MEASURE_WITH_UNIT(LENGTH_MEASURE(0.01),#130911,
'DISTANCE_ACCURACY_VALUE',
'Maximum model space distance between geometric entities at asserted c
onnectivities');
#130906=(
GEOMETRIC_REPRESENTATION_CONTEXT(3)
GLOBAL_UNCERTAINTY_ASSIGNED_CONTEXT((#130896))
GLOBAL_UNIT_ASSIGNED_CONTEXT((#130911,#130913,#130914))
REPRESENTATION_CONTEXT('','3D')
);
#130910=(
GEOMETRIC_REPRESENTATION_CONTEXT(3)
GLOBAL_UNCERTAINTY_ASSIGNED_CONTEXT((#130900))
GLOBAL_UNIT_ASSIGNED_CONTEXT((#130911,#130913,#130914))
REPRESENTATION_CONTEXT('','3D')
);
#130911=(
LENGTH_UNIT()
NAMED_UNIT(*)
SI_UNIT(.MILLI.,.METRE.)
);
#130913=(
NAMED_UNIT(*)
PLANE_ANGLE_UNIT()
SI_UNIT($,.RADIAN.)
);
#130914=(
NAMED_UNIT(*)
SI_UNIT($,.STERADIAN.)
SOLID_ANGLE_UNIT()
);
#130920=SHAPE_DEFINITION_REPRESENTATION(#130929,#130946);
#130929=PRODUCT_DEFINITION_SHAPE('',$,#130956);
#130946=SHAPE_REPRESENTATION('',(#48574),#130906);
#130950=PRODUCT_DEFINITION_CONTEXT('part definition',#130979,'design');
#130956=PRODUCT_DEFINITION('Component5','Component5',#130965,#130950);
#130965=PRODUCT_DEFINITION_FORMATION('',$,#130986);
#130979=APPLICATION_CONTEXT(
'Core Data for Automotive Mechanical Design Process');
#130980=PRODUCT_CONTEXT('part definition',#130979,'mechanical');
#130986=PRODUCT('Component5','Component5',$,(#130980));
#130991=PRESENTATION_STYLE_ASSIGNMENT((#130993));
#130993=SURFACE_STYLE_USAGE(.BOTH.,#130995);
#130995=SURFACE_SIDE_STYLE('',(#130997));
#130997=SURFACE_STYLE_FILL_AREA(#130999);
#130999=FILL_AREA_STYLE('Opaque(202,209,238)',(#131001));
#131001=FILL_AREA_STYLE_COLOUR('Opaque(202,209,238)',#131003);
#131003=COLOUR_RGB('Opaque(202,209,238)', 0.40784314, 0.44705882, 0.49803922);
ENDSEC;
END-ISO-10303-21;
